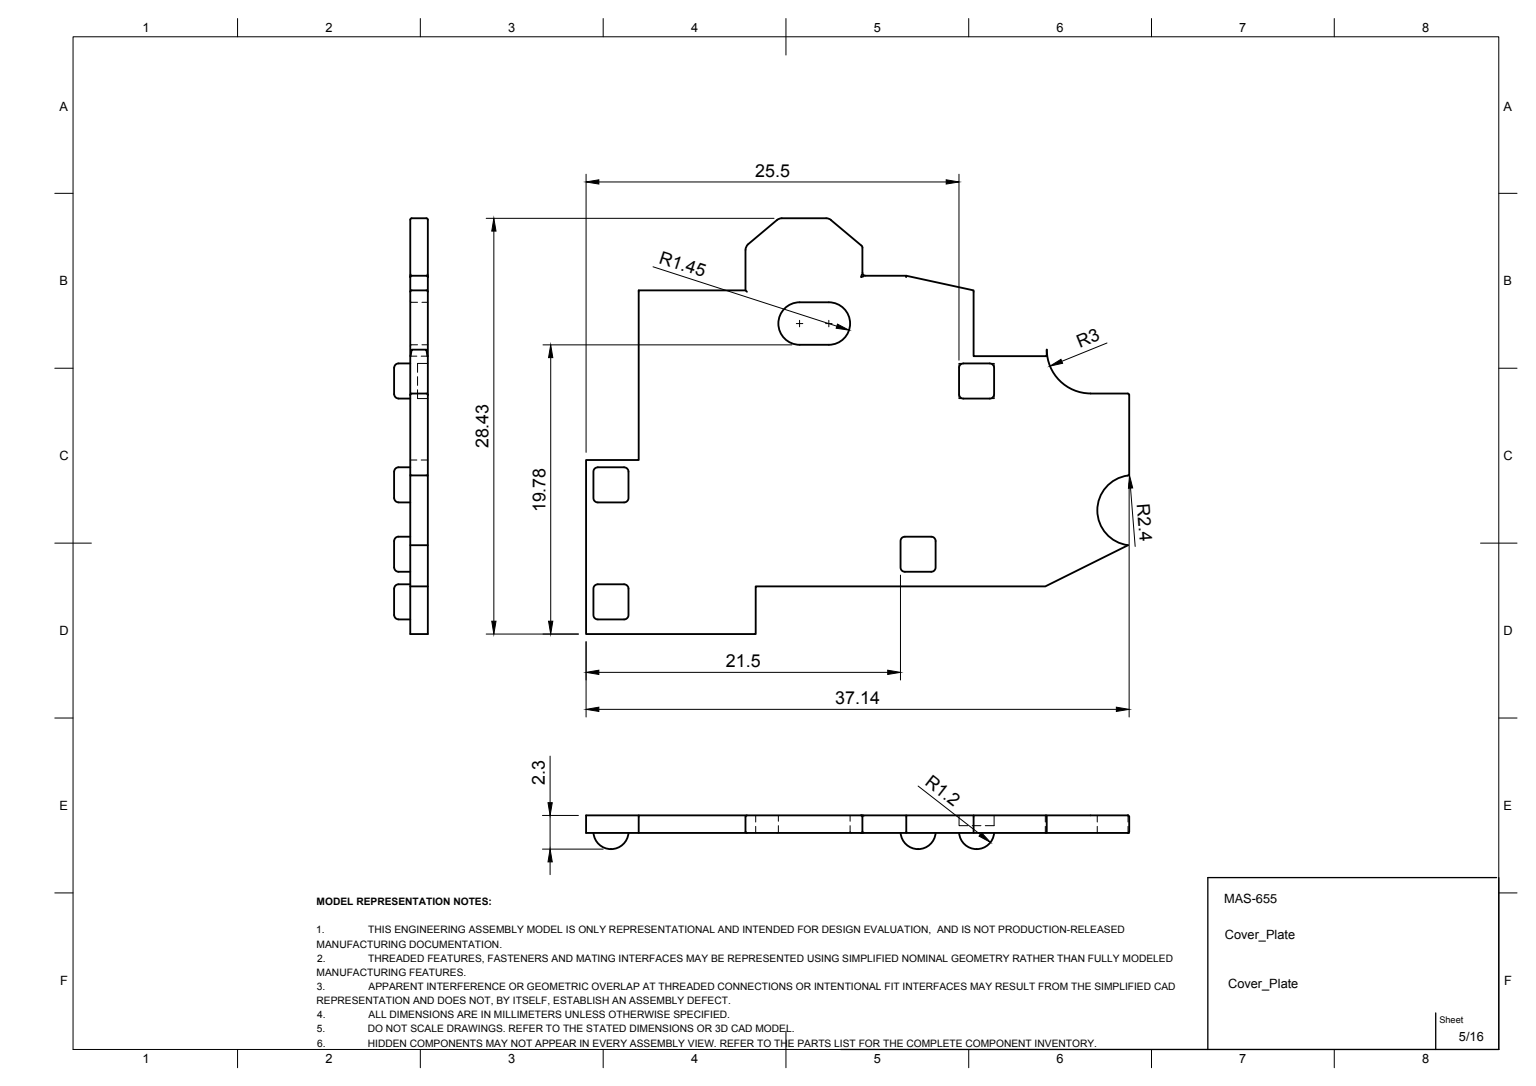
ISO-10303-21;
HEADER;
FILE_DESCRIPTION((''),'2;1');
FILE_NAME('Cover_Plate.step','2026-10-09T11:34:15-07:00',(''),(''),'','','');
FILE_SCHEMA (('AUTOMOTIVE_DESIGN { 1 0 10303 214 3 1 1 }'));
ENDSEC;
DATA;
#10=MECHANICAL_DESIGN_GEOMETRIC_PRESENTATION_REPRESENTATION('',(#632),#117170);
#95=(
BOUNDED_SURFACE()
B_SPLINE_SURFACE(2,2,((#87159,#87160,#87161),(#87162,#87163,#87164),(#87165,
#87166,#87167)),.UNSPECIFIED.,.F.,.F.,.F.)
B_SPLINE_SURFACE_WITH_KNOTS((3,3),(3,3),(2.9656421913598E-12,1.57079632680175),
(-2.44346095279454,-1.57079632680019),.UNSPECIFIED.)
GEOMETRIC_REPRESENTATION_ITEM()
RATIONAL_B_SPLINE_SURFACE(((1.,0.906307787037244,1.),(0.707106781185325,
0.640856382055101,0.707106781185325),(1.,0.906307787037244,1.)))
REPRESENTATION_ITEM('')
SURFACE()
) ;
#96=(
BOUNDED_SURFACE()
B_SPLINE_SURFACE(2,2,((#87171,#87172,#87173),(#87174,#87175,#87176),(#87177,
#87178,#87179)),.UNSPECIFIED.,.F.,.F.,.F.)
B_SPLINE_SURFACE_WITH_KNOTS((3,3),(3,3),(-1.5707963267996,-4.58626074717158E-12),
(-2.44346095281538,-1.57079632678052),.UNSPECIFIED.)
GEOMETRIC_REPRESENTATION_ITEM()
RATIONAL_B_SPLINE_SURFACE(((1.,0.906307787028686,1.),(0.707106781186676,
0.640856382050274,0.707106781186676),(1.,0.906307787028686,1.)))
REPRESENTATION_ITEM('')
SURFACE()
) ;
#269=ELLIPSE('',#51771,0.141421356237322,0.1) ;
#270=ELLIPSE('',#51774,0.141421356237322,0.1) ;
#271=ELLIPSE('',#51814,0.31622776601682,0.0999999999999979) ;
#272=ELLIPSE('',#51815,0.31622776601682,0.0999999999999979) ;
#273=ELLIPSE('',#51816,0.316227766016848,0.0999999999999979) ;
#274=ELLIPSE('',#51817,0.316227766016848,0.0999999999999979) ;
#275=ELLIPSE('',#51820,0.316227766016848,0.0999999999999979) ;
#276=ELLIPSE('',#51821,0.316227766016848,0.0999999999999979) ;
#277=ELLIPSE('',#51822,0.316227766016837,0.0999999999999979) ;
#278=ELLIPSE('',#51823,0.316227766016837,0.0999999999999979) ;
#279=ELLIPSE('',#51826,0.100574612243464,0.1) ;
#280=ELLIPSE('',#51856,0.102331928648948,0.1) ;
#281=ELLIPSE('',#51857,0.10057461224346,0.1) ;
#282=ELLIPSE('',#51862,0.102331928648948,0.1) ;
#590=SHAPE_REPRESENTATION_RELATIONSHIP('SRR','None',#117245,#611) ;
#611=ADVANCED_BREP_SHAPE_REPRESENTATION('',(#653),#117153) ;
#632=STYLED_ITEM('',(#117355),#653) ;
#653=MANIFOLD_SOLID_BREP('Body1',#49061) ;
#722=FACE_BOUND('',#15126,.T.) ;
#723=FACE_BOUND('',#15127,.T.) ;
#724=FACE_BOUND('',#15128,.T.) ;
#725=FACE_BOUND('',#15129,.T.) ;
#726=FACE_BOUND('',#15130,.T.) ;
#727=FACE_BOUND('',#15135,.T.) ;
#728=FACE_BOUND('',#15136,.T.) ;
#1127=B_SPLINE_CURVE_WITH_KNOTS('',3,(#86615,#86616,#86617,#86618,#86619,
#86620,#86621,#86622,#86623,#86624),.UNSPECIFIED.,.F.,.F.,(4,2,2,2,4),(-0.0453895164641597,
-0.0415954731675521,-0.0378014298709444,-0.0340366298274179,-0.0302718297838914),
 .UNSPECIFIED.) ;
#1128=B_SPLINE_CURVE_WITH_KNOTS('',3,(#86641,#86642,#86643,#86644,#86645,
#86646,#86647,#86648,#86649,#86650),.UNSPECIFIED.,.F.,.F.,(4,2,2,2,4),(-0.0302718297838915,
-0.0265011188029211,-0.0227304078219508,-0.0189422746940918,-0.0151541415662328),
 .UNSPECIFIED.) ;
#1129=B_SPLINE_CURVE_WITH_KNOTS('',3,(#86717,#86718,#86719,#86720,#86721,
#86722,#86723,#86724,#86725,#86726),.UNSPECIFIED.,.F.,.F.,(4,2,2,2,4),(0.13378524314305,
0.14497374491656,0.1561177263117,0.167229804836174,0.17832206951723),
 .UNSPECIFIED.) ;
#1130=B_SPLINE_CURVE_WITH_KNOTS('',3,(#86730,#86731,#86732,#86733,#86734,
#86735,#86736,#86737,#86738,#86739),.UNSPECIFIED.,.F.,.F.,(4,2,2,2,4),(0.,
0.0110922646810569,0.0222043432055302,0.0333483246006708,0.0445368263741803),
 .UNSPECIFIED.) ;
#1131=B_SPLINE_CURVE_WITH_KNOTS('',3,(#86743,#86744,#86745,#86746,#86747,
#86748,#86749,#86750,#86751,#86752),.UNSPECIFIED.,.F.,.F.,(4,2,2,2,4),(0.13378524314305,
0.14497374491656,0.1561177263117,0.167229804836174,0.17832206951723),
 .UNSPECIFIED.) ;
#1132=B_SPLINE_CURVE_WITH_KNOTS('',3,(#86756,#86757,#86758,#86759,#86760,
#86761,#86762,#86763,#86764,#86765),.UNSPECIFIED.,.F.,.F.,(4,2,2,2,4),(0.,
0.0110922646810569,0.0222043432055302,0.0333483246006708,0.0445368263741803),
 .UNSPECIFIED.) ;
#1133=B_SPLINE_CURVE_WITH_KNOTS('',3,(#86771,#86772,#86773,#86774,#86775,
#86776,#86777,#86778,#86779,#86780),.UNSPECIFIED.,.F.,.F.,(4,2,2,2,4),(0.,
0.0110922646810569,0.0222043432055302,0.0333483246006708,0.0445368263741803),
 .UNSPECIFIED.) ;
#1134=B_SPLINE_CURVE_WITH_KNOTS('',3,(#86784,#86785,#86786,#86787,#86788,
#86789,#86790,#86791,#86792,#86793),.UNSPECIFIED.,.F.,.F.,(4,2,2,2,4),(0.133785243143047,
0.144973744916557,0.156117726311698,0.167229804836173,0.17832206951723),
 .UNSPECIFIED.) ;
#1135=B_SPLINE_CURVE_WITH_KNOTS('',3,(#86797,#86798,#86799,#86800,#86801,
#86802,#86803,#86804,#86805,#86806),.UNSPECIFIED.,.F.,.F.,(4,2,2,2,4),(0.,
0.0110922646810577,0.022204343205532,0.0333483246006734,0.0445368263741838),
 .UNSPECIFIED.) ;
#1136=B_SPLINE_CURVE_WITH_KNOTS('',3,(#86809,#86810,#86811,#86812,#86813,
#86814,#86815,#86816,#86817,#86818),.UNSPECIFIED.,.F.,.F.,(4,2,2,2,4),(0.13378524314305,
0.14497374491656,0.1561177263117,0.167229804836174,0.17832206951723),
 .UNSPECIFIED.) ;
#1137=B_SPLINE_CURVE_WITH_KNOTS('',3,(#86823,#86824,#86825,#86826,#86827,
#86828,#86829,#86830,#86831,#86832),.UNSPECIFIED.,.F.,.F.,(4,2,2,2,4),(0.,
0.0110922646810577,0.022204343205532,0.0333483246006734,0.0445368263741838),
 .UNSPECIFIED.) ;
#1138=B_SPLINE_CURVE_WITH_KNOTS('',3,(#86836,#86837,#86838,#86839,#86840,
#86841,#86842,#86843,#86844,#86845),.UNSPECIFIED.,.F.,.F.,(4,2,2,2,4),(0.13378524314305,
0.14497374491656,0.1561177263117,0.167229804836174,0.17832206951723),
 .UNSPECIFIED.) ;
#1139=B_SPLINE_CURVE_WITH_KNOTS('',3,(#86849,#86850,#86851,#86852,#86853,
#86854,#86855,#86856,#86857,#86858),.UNSPECIFIED.,.F.,.F.,(4,2,2,2,4),(0.,
0.0110922646810569,0.0222043432055302,0.0333483246006708,0.0445368263741803),
 .UNSPECIFIED.) ;
#1140=B_SPLINE_CURVE_WITH_KNOTS('',3,(#86861,#86862,#86863,#86864,#86865,
#86866,#86867,#86868,#86869,#86870),.UNSPECIFIED.,.F.,.F.,(4,2,2,2,4),(0.133785243143047,
0.144973744916557,0.156117726311698,0.167229804836173,0.17832206951723),
 .UNSPECIFIED.) ;
#1141=B_SPLINE_CURVE_WITH_KNOTS('',3,(#86875,#86876,#86877,#86878,#86879,
#86880,#86881,#86882,#86883,#86884),.UNSPECIFIED.,.F.,.F.,(4,2,2,2,4),(0.,
0.0110922646810569,0.0222043432055302,0.0333483246006708,0.0445368263741803),
 .UNSPECIFIED.) ;
#1142=B_SPLINE_CURVE_WITH_KNOTS('',3,(#86888,#86889,#86890,#86891,#86892,
#86893,#86894,#86895,#86896,#86897),.UNSPECIFIED.,.F.,.F.,(4,2,2,2,4),(0.133785243143047,
0.144973744916557,0.156117726311698,0.167229804836173,0.17832206951723),
 .UNSPECIFIED.) ;
#1143=B_SPLINE_CURVE_WITH_KNOTS('',3,(#86901,#86902,#86903,#86904,#86905,
#86906,#86907,#86908,#86909,#86910),.UNSPECIFIED.,.F.,.F.,(4,2,2,2,4),(0.,
0.0110922646810577,0.022204343205532,0.0333483246006734,0.0445368263741838),
 .UNSPECIFIED.) ;
#1144=B_SPLINE_CURVE_WITH_KNOTS('',3,(#86913,#86914,#86915,#86916,#86917,
#86918,#86919,#86920,#86921,#86922),.UNSPECIFIED.,.F.,.F.,(4,2,2,2,4),(0.13378524314305,
0.14497374491656,0.1561177263117,0.167229804836174,0.17832206951723),
 .UNSPECIFIED.) ;
#1145=B_SPLINE_CURVE_WITH_KNOTS('',3,(#87209,#87210,#87211,#87212,#87213,
#87214),.UNSPECIFIED.,.F.,.F.,(4,2,4),(0.0376778444829456,0.0409098759506884,
0.0446641096906363),.UNSPECIFIED.) ;
#1146=B_SPLINE_CURVE_WITH_KNOTS('',3,(#87217,#87218,#87219,#87220),
 .UNSPECIFIED.,.F.,.F.,(4,4),(0.,0.0422101666362959),.UNSPECIFIED.) ;
#1147=B_SPLINE_CURVE_WITH_KNOTS('',3,(#87225,#87226,#87227,#87228),
 .UNSPECIFIED.,.F.,.F.,(4,4),(-0.0422101666362958,0.),.UNSPECIFIED.) ;
#1148=B_SPLINE_CURVE_WITH_KNOTS('',3,(#87235,#87236,#87237,#87238,#87239,
#87240),.UNSPECIFIED.,.F.,.F.,(4,2,4),(0.0148851463516941,0.0186393800916421,
0.021871411559383),.UNSPECIFIED.) ;
#1989=B_SPLINE_SURFACE_WITH_KNOTS('',3,3,((#87076,#87077,#87078,#87079,
#87080),(#87081,#87082,#87083,#87084,#87085),(#87086,#87087,#87088,#87089,
#87090),(#87091,#87092,#87093,#87094,#87095),(#87096,#87097,#87098,#87099,
#87100)),.UNSPECIFIED.,.F.,.F.,.F.,(4,1,4),(4,1,4),(-0.000337535876093274,
0.5,1.00033753587942),(-1.5707963267949,-0.897597901025655,0.000337535879419949),
 .UNSPECIFIED.) ;
#1990=B_SPLINE_SURFACE_WITH_KNOTS('',3,3,((#87116,#87117,#87118,#87119,
#87120),(#87121,#87122,#87123,#87124,#87125),(#87126,#87127,#87128,#87129,
#87130),(#87131,#87132,#87133,#87134,#87135),(#87136,#87137,#87138,#87139,
#87140)),.UNSPECIFIED.,.F.,.F.,.F.,(4,1,4),(4,1,4),(-0.000337608092631786,
0.5,1.00033760812633),(-1.5707963267949,-0.897597901025655,0.000337608126388777),
 .UNSPECIFIED.) ;
#2193=SPHERICAL_SURFACE('',#51742,0.1) ;
#2194=SPHERICAL_SURFACE('',#51744,0.1) ;
#2435=PLANE('',#51746) ;
#2436=PLANE('',#51757) ;
#2437=PLANE('',#51760) ;
#2438=PLANE('',#51775) ;
#2439=PLANE('',#51785) ;
#2440=PLANE('',#51799) ;
#2441=PLANE('',#51810) ;
#2442=PLANE('',#51824) ;
#2443=PLANE('',#51834) ;
#2444=PLANE('',#51846) ;
#2445=PLANE('',#51849) ;
#2446=PLANE('',#51852) ;
#2447=PLANE('',#51854) ;
#2448=PLANE('',#51861) ;
#2449=PLANE('',#51863) ;
#2450=PLANE('',#51864) ;
#2451=PLANE('',#51876) ;
#2452=PLANE('',#51886) ;
#2453=PLANE('',#51896) ;
#2454=PLANE('',#51906) ;
#2455=PLANE('',#51916) ;
#2456=PLANE('',#51926) ;
#2457=PLANE('',#51936) ;
#2458=PLANE('',#51946) ;
#2459=PLANE('',#51948) ;
#2460=PLANE('',#51951) ;
#2461=PLANE('',#51954) ;
#2462=PLANE('',#51957) ;
#2463=PLANE('',#51959) ;
#2464=PLANE('',#51960) ;
#2465=PLANE('',#51961) ;
#2466=PLANE('',#51963) ;
#2467=PLANE('',#51964) ;
#2468=PLANE('',#51966) ;
#2469=PLANE('',#51967) ;
#2470=PLANE('',#51968) ;
#2471=PLANE('',#51969) ;
#2472=PLANE('',#51970) ;
#2473=PLANE('',#51971) ;
#2474=PLANE('',#51972) ;
#2475=PLANE('',#51973) ;
#4105=LINE('',#86626,#7319) ;
#4106=LINE('',#86629,#7320) ;
#4107=LINE('',#86634,#7321) ;
#4108=LINE('',#86637,#7322) ;
#4109=LINE('',#86652,#7323) ;
#4110=LINE('',#86654,#7324) ;
#4111=LINE('',#86661,#7325) ;
#4112=LINE('',#86665,#7326) ;
#4113=LINE('',#86667,#7327) ;
#4114=LINE('',#86669,#7328) ;
#4115=LINE('',#86671,#7329) ;
#4116=LINE('',#86673,#7330) ;
#4117=LINE('',#86677,#7331) ;
#4118=LINE('',#86681,#7332) ;
#4119=LINE('',#86685,#7333) ;
#4120=LINE('',#86689,#7334) ;
#4121=LINE('',#86691,#7335) ;
#4122=LINE('',#86693,#7336) ;
#4123=LINE('',#86695,#7337) ;
#4124=LINE('',#86697,#7338) ;
#4125=LINE('',#86699,#7339) ;
#4126=LINE('',#86701,#7340) ;
#4127=LINE('',#86703,#7341) ;
#4128=LINE('',#86705,#7342) ;
#4129=LINE('',#86709,#7343) ;
#4130=LINE('',#86713,#7344) ;
#4131=LINE('',#86728,#7345) ;
#4132=LINE('',#86741,#7346) ;
#4133=LINE('',#86754,#7347) ;
#4134=LINE('',#86766,#7348) ;
#4135=LINE('',#86769,#7349) ;
#4136=LINE('',#86782,#7350) ;
#4137=LINE('',#86795,#7351) ;
#4138=LINE('',#86808,#7352) ;
#4139=LINE('',#86821,#7353) ;
#4140=LINE('',#86834,#7354) ;
#4141=LINE('',#86847,#7355) ;
#4142=LINE('',#86860,#7356) ;
#4143=LINE('',#86873,#7357) ;
#4144=LINE('',#86886,#7358) ;
#4145=LINE('',#86899,#7359) ;
#4146=LINE('',#86912,#7360) ;
#4147=LINE('',#86925,#7361) ;
#4148=LINE('',#86929,#7362) ;
#4149=LINE('',#86930,#7363) ;
#4150=LINE('',#86933,#7364) ;
#4151=LINE('',#86939,#7365) ;
#4152=LINE('',#86941,#7366) ;
#4153=LINE('',#86943,#7367) ;
#4154=LINE('',#86945,#7368) ;
#4155=LINE('',#86947,#7369) ;
#4156=LINE('',#86949,#7370) ;
#4157=LINE('',#86951,#7371) ;
#4158=LINE('',#86953,#7372) ;
#4159=LINE('',#86955,#7373) ;
#4160=LINE('',#86959,#7374) ;
#4161=LINE('',#86963,#7375) ;
#4162=LINE('',#86967,#7376) ;
#4163=LINE('',#86971,#7377) ;
#4164=LINE('',#86973,#7378) ;
#4165=LINE('',#86975,#7379) ;
#4166=LINE('',#86977,#7380) ;
#4167=LINE('',#86979,#7381) ;
#4168=LINE('',#86985,#7382) ;
#4169=LINE('',#86988,#7383) ;
#4170=LINE('',#86991,#7384) ;
#4171=LINE('',#86993,#7385) ;
#4172=LINE('',#86995,#7386) ;
#4173=LINE('',#86996,#7387) ;
#4174=LINE('',#87001,#7388) ;
#4175=LINE('',#87008,#7389) ;
#4176=LINE('',#87010,#7390) ;
#4177=LINE('',#87011,#7391) ;
#4178=LINE('',#87025,#7392) ;
#4179=LINE('',#87026,#7393) ;
#4180=LINE('',#87029,#7394) ;
#4181=LINE('',#87031,#7395) ;
#4182=LINE('',#87032,#7396) ;
#4183=LINE('',#87037,#7397) ;
#4184=LINE('',#87050,#7398) ;
#4185=LINE('',#87051,#7399) ;
#4186=LINE('',#87053,#7400) ;
#4187=LINE('',#87065,#7401) ;
#4188=LINE('',#87068,#7402) ;
#4189=LINE('',#87072,#7403) ;
#4190=LINE('',#87073,#7404) ;
#4191=LINE('',#87112,#7405) ;
#4192=LINE('',#87115,#7406) ;
#4193=LINE('',#87149,#7407) ;
#4194=LINE('',#87151,#7408) ;
#4195=LINE('',#87152,#7409) ;
#4196=LINE('',#87157,#7410) ;
#4197=LINE('',#87182,#7411) ;
#4198=LINE('',#87184,#7412) ;
#4199=LINE('',#87191,#7413) ;
#4200=LINE('',#87199,#7414) ;
#4201=LINE('',#87203,#7415) ;
#4202=LINE('',#87204,#7416) ;
#4203=LINE('',#87206,#7417) ;
#4204=LINE('',#87223,#7418) ;
#4205=LINE('',#87229,#7419) ;
#4206=LINE('',#87233,#7420) ;
#4207=LINE('',#87242,#7421) ;
#4208=LINE('',#87245,#7422) ;
#4209=LINE('',#87251,#7423) ;
#4210=LINE('',#87254,#7424) ;
#4211=LINE('',#87257,#7425) ;
#4212=LINE('',#87259,#7426) ;
#4213=LINE('',#87272,#7427) ;
#4214=LINE('',#87273,#7428) ;
#4215=LINE('',#87288,#7429) ;
#4216=LINE('',#87289,#7430) ;
#4217=LINE('',#87304,#7431) ;
#4218=LINE('',#87305,#7432) ;
#4219=LINE('',#87320,#7433) ;
#4220=LINE('',#87321,#7434) ;
#4221=LINE('',#87336,#7435) ;
#4222=LINE('',#87337,#7436) ;
#4223=LINE('',#87352,#7437) ;
#4224=LINE('',#87353,#7438) ;
#4225=LINE('',#87368,#7439) ;
#4226=LINE('',#87369,#7440) ;
#4227=LINE('',#87384,#7441) ;
#4228=LINE('',#87385,#7442) ;
#4229=LINE('',#87391,#7443) ;
#4230=LINE('',#87393,#7444) ;
#4231=LINE('',#87396,#7445) ;
#4232=LINE('',#87398,#7446) ;
#4233=LINE('',#87401,#7447) ;
#4234=LINE('',#87403,#7448) ;
#4235=LINE('',#87406,#7449) ;
#4236=LINE('',#87408,#7450) ;
#4237=LINE('',#87413,#7451) ;
#4238=LINE('',#87415,#7452) ;
#4239=LINE('',#87417,#7453) ;
#4240=LINE('',#87418,#7454) ;
#4241=LINE('',#87420,#7455) ;
#4242=LINE('',#87421,#7456) ;
#4243=LINE('',#87423,#7457) ;
#4244=LINE('',#87425,#7458) ;
#4245=LINE('',#87427,#7459) ;
#4246=LINE('',#87429,#7460) ;
#4247=LINE('',#87432,#7461) ;
#4248=LINE('',#87435,#7462) ;
#4249=LINE('',#87437,#7463) ;
#4250=LINE('',#87439,#7464) ;
#4251=LINE('',#87441,#7465) ;
#4252=LINE('',#87443,#7466) ;
#7319=VECTOR('',#61022,10.) ;
#7320=VECTOR('',#61025,10.) ;
#7321=VECTOR('',#61030,10.) ;
#7322=VECTOR('',#61033,10.) ;
#7323=VECTOR('',#61036,10.) ;
#7324=VECTOR('',#61039,10.) ;
#7325=VECTOR('',#61050,10.) ;
#7326=VECTOR('',#61053,10.) ;
#7327=VECTOR('',#61054,10.) ;
#7328=VECTOR('',#61055,10.) ;
#7329=VECTOR('',#61056,10.) ;
#7330=VECTOR('',#61057,10.) ;
#7331=VECTOR('',#61060,10.) ;
#7332=VECTOR('',#61063,10.) ;
#7333=VECTOR('',#61066,10.) ;
#7334=VECTOR('',#61069,10.) ;
#7335=VECTOR('',#61070,10.) ;
#7336=VECTOR('',#61071,10.) ;
#7337=VECTOR('',#61072,10.) ;
#7338=VECTOR('',#61073,10.) ;
#7339=VECTOR('',#61074,10.) ;
#7340=VECTOR('',#61075,10.) ;
#7341=VECTOR('',#61076,10.) ;
#7342=VECTOR('',#61077,10.) ;
#7343=VECTOR('',#61080,10.) ;
#7344=VECTOR('',#61083,10.) ;
#7345=VECTOR('',#61086,10.) ;
#7346=VECTOR('',#61087,10.) ;
#7347=VECTOR('',#61088,10.) ;
#7348=VECTOR('',#61089,10.) ;
#7349=VECTOR('',#61090,10.) ;
#7350=VECTOR('',#61091,10.) ;
#7351=VECTOR('',#61092,10.) ;
#7352=VECTOR('',#61093,10.) ;
#7353=VECTOR('',#61094,10.) ;
#7354=VECTOR('',#61095,10.) ;
#7355=VECTOR('',#61096,10.) ;
#7356=VECTOR('',#61097,10.) ;
#7357=VECTOR('',#61098,10.) ;
#7358=VECTOR('',#61099,10.) ;
#7359=VECTOR('',#61100,10.) ;
#7360=VECTOR('',#61101,10.) ;
#7361=VECTOR('',#61104,10.) ;
#7362=VECTOR('',#61109,10.) ;
#7363=VECTOR('',#61110,10.) ;
#7364=VECTOR('',#61113,10.) ;
#7365=VECTOR('',#61120,10.) ;
#7366=VECTOR('',#61121,10.) ;
#7367=VECTOR('',#61122,10.) ;
#7368=VECTOR('',#61123,10.) ;
#7369=VECTOR('',#61124,10.) ;
#7370=VECTOR('',#61125,10.) ;
#7371=VECTOR('',#61126,10.) ;
#7372=VECTOR('',#61127,10.) ;
#7373=VECTOR('',#61128,10.) ;
#7374=VECTOR('',#61131,10.) ;
#7375=VECTOR('',#61134,10.) ;
#7376=VECTOR('',#61137,10.) ;
#7377=VECTOR('',#61140,10.) ;
#7378=VECTOR('',#61141,10.) ;
#7379=VECTOR('',#61142,10.) ;
#7380=VECTOR('',#61143,10.) ;
#7381=VECTOR('',#61144,10.) ;
#7382=VECTOR('',#61149,10.) ;
#7383=VECTOR('',#61152,10.) ;
#7384=VECTOR('',#61153,10.) ;
#7385=VECTOR('',#61154,10.) ;
#7386=VECTOR('',#61155,10.) ;
#7387=VECTOR('',#61156,10.) ;
#7388=VECTOR('',#61161,10.) ;
#7389=VECTOR('',#61170,10.) ;
#7390=VECTOR('',#61173,10.) ;
#7391=VECTOR('',#61174,10.) ;
#7392=VECTOR('',#61193,10.) ;
#7393=VECTOR('',#61194,10.) ;
#7394=VECTOR('',#61197,10.) ;
#7395=VECTOR('',#61198,10.) ;
#7396=VECTOR('',#61199,10.) ;
#7397=VECTOR('',#61206,10.) ;
#7398=VECTOR('',#61225,10.) ;
#7399=VECTOR('',#61226,10.) ;
#7400=VECTOR('',#61229,10.) ;
#7401=VECTOR('',#61248,10.) ;
#7402=VECTOR('',#61251,10.) ;
#7403=VECTOR('',#61256,10.) ;
#7404=VECTOR('',#61257,10.) ;
#7405=VECTOR('',#61274,10.) ;
#7406=VECTOR('',#61277,10.) ;
#7407=VECTOR('',#61288,10.) ;
#7408=VECTOR('',#61289,10.) ;
#7409=VECTOR('',#61290,10.) ;
#7410=VECTOR('',#61297,10.) ;
#7411=VECTOR('',#61308,10.) ;
#7412=VECTOR('',#61311,10.) ;
#7413=VECTOR('',#61320,10.) ;
#7414=VECTOR('',#61331,10.) ;
#7415=VECTOR('',#61338,10.) ;
#7416=VECTOR('',#61339,10.) ;
#7417=VECTOR('',#61342,10.) ;
#7418=VECTOR('',#61349,10.) ;
#7419=VECTOR('',#61350,10.) ;
#7420=VECTOR('',#61357,10.) ;
#7421=VECTOR('',#61362,10.) ;
#7422=VECTOR('',#61365,10.) ;
#7423=VECTOR('',#61376,10.) ;
#7424=VECTOR('',#61379,10.) ;
#7425=VECTOR('',#61384,10.) ;
#7426=VECTOR('',#61387,10.) ;
#7427=VECTOR('',#61404,10.) ;
#7428=VECTOR('',#61405,10.) ;
#7429=VECTOR('',#61426,10.) ;
#7430=VECTOR('',#61427,10.) ;
#7431=VECTOR('',#61448,10.) ;
#7432=VECTOR('',#61449,10.) ;
#7433=VECTOR('',#61470,10.) ;
#7434=VECTOR('',#61471,10.) ;
#7435=VECTOR('',#61492,10.) ;
#7436=VECTOR('',#61493,10.) ;
#7437=VECTOR('',#61514,10.) ;
#7438=VECTOR('',#61515,10.) ;
#7439=VECTOR('',#61536,10.) ;
#7440=VECTOR('',#61537,10.) ;
#7441=VECTOR('',#61558,10.) ;
#7442=VECTOR('',#61559,10.) ;
#7443=VECTOR('',#61570,1.2) ;
#7444=VECTOR('',#61573,1.2) ;
#7445=VECTOR('',#61578,1.2) ;
#7446=VECTOR('',#61581,1.2) ;
#7447=VECTOR('',#61586,1.2) ;
#7448=VECTOR('',#61589,1.2) ;
#7449=VECTOR('',#61594,1.2) ;
#7450=VECTOR('',#61597,1.2) ;
#7451=VECTOR('',#61602,10.) ;
#7452=VECTOR('',#61603,10.) ;
#7453=VECTOR('',#61604,10.) ;
#7454=VECTOR('',#61605,10.) ;
#7455=VECTOR('',#61608,10.) ;
#7456=VECTOR('',#61609,10.) ;
#7457=VECTOR('',#61612,10.) ;
#7458=VECTOR('',#61615,10.) ;
#7459=VECTOR('',#61618,10.) ;
#7460=VECTOR('',#61621,10.) ;
#7461=VECTOR('',#61626,10.) ;
#7462=VECTOR('',#61631,10.) ;
#7463=VECTOR('',#61634,10.) ;
#7464=VECTOR('',#61637,10.) ;
#7465=VECTOR('',#61640,10.) ;
#7466=VECTOR('',#61643,10.) ;
#9939=CYLINDRICAL_SURFACE('',#51735,0.1) ;
#9940=CYLINDRICAL_SURFACE('',#51737,0.1) ;
#9941=CYLINDRICAL_SURFACE('',#51740,0.1) ;
#9942=CYLINDRICAL_SURFACE('',#51755,0.1) ;
#9943=CYLINDRICAL_SURFACE('',#51758,0.1) ;
#9944=CYLINDRICAL_SURFACE('',#51769,0.1) ;
#9945=CYLINDRICAL_SURFACE('',#51772,0.1) ;
#9946=CYLINDRICAL_SURFACE('',#51784,0.5) ;
#9947=CYLINDRICAL_SURFACE('',#51786,0.1) ;
#9948=CYLINDRICAL_SURFACE('',#51788,0.1) ;
#9949=CYLINDRICAL_SURFACE('',#51797,0.5) ;
#9950=CYLINDRICAL_SURFACE('',#51798,0.1) ;
#9951=CYLINDRICAL_SURFACE('',#51807,0.5) ;
#9952=CYLINDRICAL_SURFACE('',#51808,0.1) ;
#9953=CYLINDRICAL_SURFACE('',#51811,0.1) ;
#9954=CYLINDRICAL_SURFACE('',#51818,0.2) ;
#9955=CYLINDRICAL_SURFACE('',#51825,0.1) ;
#9956=CYLINDRICAL_SURFACE('',#51827,0.1) ;
#9957=CYLINDRICAL_SURFACE('',#51832,0.2) ;
#9958=CYLINDRICAL_SURFACE('',#51833,0.1) ;
#9959=CYLINDRICAL_SURFACE('',#51835,0.1) ;
#9960=CYLINDRICAL_SURFACE('',#51841,0.1) ;
#9961=CYLINDRICAL_SURFACE('',#51845,1.45266329058736) ;
#9962=CYLINDRICAL_SURFACE('',#51850,3.) ;
#9963=CYLINDRICAL_SURFACE('',#51855,0.1) ;
#9964=CYLINDRICAL_SURFACE('',#51858,0.1) ;
#9965=CYLINDRICAL_SURFACE('',#51859,0.1) ;
#9966=CYLINDRICAL_SURFACE('',#51860,0.1) ;
#9967=CYLINDRICAL_SURFACE('',#51865,0.1) ;
#9968=CYLINDRICAL_SURFACE('',#51866,0.1) ;
#9969=CYLINDRICAL_SURFACE('',#51871,0.3) ;
#9970=CYLINDRICAL_SURFACE('',#51881,0.3) ;
#9971=CYLINDRICAL_SURFACE('',#51891,0.3) ;
#9972=CYLINDRICAL_SURFACE('',#51901,0.3) ;
#9973=CYLINDRICAL_SURFACE('',#51911,0.3) ;
#9974=CYLINDRICAL_SURFACE('',#51921,0.3) ;
#9975=CYLINDRICAL_SURFACE('',#51931,0.3) ;
#9976=CYLINDRICAL_SURFACE('',#51941,0.3) ;
#9977=CYLINDRICAL_SURFACE('',#51947,1.19999999999999) ;
#9978=CYLINDRICAL_SURFACE('',#51949,1.19999999999999) ;
#9979=CYLINDRICAL_SURFACE('',#51950,1.19999999999999) ;
#9980=CYLINDRICAL_SURFACE('',#51952,1.19999999999999) ;
#9981=CYLINDRICAL_SURFACE('',#51953,1.19999999999999) ;
#9982=CYLINDRICAL_SURFACE('',#51955,1.19999999999999) ;
#9983=CYLINDRICAL_SURFACE('',#51956,1.19999999999999) ;
#9984=CYLINDRICAL_SURFACE('',#51958,1.19999999999999) ;
#9985=CYLINDRICAL_SURFACE('',#51962,2.4) ;
#9986=CYLINDRICAL_SURFACE('',#51965,1.45266329058736) ;
#11976=FACE_OUTER_BOUND('',#15120,.T.) ;
#11977=FACE_OUTER_BOUND('',#15121,.T.) ;
#11978=FACE_OUTER_BOUND('',#15122,.T.) ;
#11979=FACE_OUTER_BOUND('',#15123,.T.) ;
#11980=FACE_OUTER_BOUND('',#15124,.T.) ;
#11981=FACE_OUTER_BOUND('',#15125,.T.) ;
#11982=FACE_OUTER_BOUND('',#15131,.T.) ;
#11983=FACE_OUTER_BOUND('',#15132,.T.) ;
#11984=FACE_OUTER_BOUND('',#15133,.T.) ;
#11985=FACE_OUTER_BOUND('',#15134,.T.) ;
#11986=FACE_OUTER_BOUND('',#15137,.T.) ;
#11987=FACE_OUTER_BOUND('',#15138,.T.) ;
#11988=FACE_OUTER_BOUND('',#15139,.T.) ;
#11989=FACE_OUTER_BOUND('',#15140,.T.) ;
#11990=FACE_OUTER_BOUND('',#15141,.T.) ;
#11991=FACE_OUTER_BOUND('',#15142,.T.) ;
#11992=FACE_OUTER_BOUND('',#15143,.T.) ;
#11993=FACE_OUTER_BOUND('',#15144,.T.) ;
#11994=FACE_OUTER_BOUND('',#15145,.T.) ;
#11995=FACE_OUTER_BOUND('',#15146,.T.) ;
#11996=FACE_OUTER_BOUND('',#15147,.T.) ;
#11997=FACE_OUTER_BOUND('',#15148,.T.) ;
#11998=FACE_OUTER_BOUND('',#15149,.T.) ;
#11999=FACE_OUTER_BOUND('',#15150,.T.) ;
#12000=FACE_OUTER_BOUND('',#15151,.T.) ;
#12001=FACE_OUTER_BOUND('',#15152,.T.) ;
#12002=FACE_OUTER_BOUND('',#15153,.T.) ;
#12003=FACE_OUTER_BOUND('',#15154,.T.) ;
#12004=FACE_OUTER_BOUND('',#15155,.T.) ;
#12005=FACE_OUTER_BOUND('',#15156,.T.) ;
#12006=FACE_OUTER_BOUND('',#15157,.T.) ;
#12007=FACE_OUTER_BOUND('',#15158,.T.) ;
#12008=FACE_OUTER_BOUND('',#15159,.T.) ;
#12009=FACE_OUTER_BOUND('',#15160,.T.) ;
#12010=FACE_OUTER_BOUND('',#15161,.T.) ;
#12011=FACE_OUTER_BOUND('',#15162,.T.) ;
#12012=FACE_OUTER_BOUND('',#15163,.T.) ;
#12013=FACE_OUTER_BOUND('',#15164,.T.) ;
#12014=FACE_OUTER_BOUND('',#15165,.T.) ;
#12015=FACE_OUTER_BOUND('',#15166,.T.) ;
#12016=FACE_OUTER_BOUND('',#15167,.T.) ;
#12017=FACE_OUTER_BOUND('',#15168,.T.) ;
#12018=FACE_OUTER_BOUND('',#15169,.T.) ;
#12019=FACE_OUTER_BOUND('',#15170,.T.) ;
#12020=FACE_OUTER_BOUND('',#15171,.T.) ;
#12021=FACE_OUTER_BOUND('',#15172,.T.) ;
#12022=FACE_OUTER_BOUND('',#15173,.T.) ;
#12023=FACE_OUTER_BOUND('',#15174,.T.) ;
#12024=FACE_OUTER_BOUND('',#15175,.T.) ;
#12025=FACE_OUTER_BOUND('',#15176,.T.) ;
#12026=FACE_OUTER_BOUND('',#15177,.T.) ;
#12027=FACE_OUTER_BOUND('',#15178,.T.) ;
#12028=FACE_OUTER_BOUND('',#15179,.T.) ;
#12029=FACE_OUTER_BOUND('',#15180,.T.) ;
#12030=FACE_OUTER_BOUND('',#15181,.T.) ;
#12031=FACE_OUTER_BOUND('',#15182,.T.) ;
#12032=FACE_OUTER_BOUND('',#15183,.T.) ;
#12033=FACE_OUTER_BOUND('',#15184,.T.) ;
#12034=FACE_OUTER_BOUND('',#15185,.T.) ;
#12035=FACE_OUTER_BOUND('',#15186,.T.) ;
#12036=FACE_OUTER_BOUND('',#15187,.T.) ;
#12037=FACE_OUTER_BOUND('',#15188,.T.) ;
#12038=FACE_OUTER_BOUND('',#15189,.T.) ;
#12039=FACE_OUTER_BOUND('',#15190,.T.) ;
#12040=FACE_OUTER_BOUND('',#15191,.T.) ;
#12041=FACE_OUTER_BOUND('',#15192,.T.) ;
#12042=FACE_OUTER_BOUND('',#15193,.T.) ;
#12043=FACE_OUTER_BOUND('',#15194,.T.) ;
#12044=FACE_OUTER_BOUND('',#15195,.T.) ;
#12045=FACE_OUTER_BOUND('',#15196,.T.) ;
#12046=FACE_OUTER_BOUND('',#15197,.T.) ;
#12047=FACE_OUTER_BOUND('',#15198,.T.) ;
#12048=FACE_OUTER_BOUND('',#15199,.T.) ;
#12049=FACE_OUTER_BOUND('',#15200,.T.) ;
#12050=FACE_OUTER_BOUND('',#15201,.T.) ;
#12051=FACE_OUTER_BOUND('',#15202,.T.) ;
#12052=FACE_OUTER_BOUND('',#15203,.T.) ;
#12053=FACE_OUTER_BOUND('',#15204,.T.) ;
#12054=FACE_OUTER_BOUND('',#15205,.T.) ;
#12055=FACE_OUTER_BOUND('',#15206,.T.) ;
#12056=FACE_OUTER_BOUND('',#15207,.T.) ;
#12057=FACE_OUTER_BOUND('',#15208,.T.) ;
#12058=FACE_OUTER_BOUND('',#15209,.T.) ;
#12059=FACE_OUTER_BOUND('',#15210,.T.) ;
#12060=FACE_OUTER_BOUND('',#15211,.T.) ;
#12061=FACE_OUTER_BOUND('',#15212,.T.) ;
#12062=FACE_OUTER_BOUND('',#15213,.T.) ;
#12063=FACE_OUTER_BOUND('',#15214,.T.) ;
#12064=FACE_OUTER_BOUND('',#15215,.T.) ;
#12065=FACE_OUTER_BOUND('',#15216,.T.) ;
#12066=FACE_OUTER_BOUND('',#15217,.T.) ;
#12067=FACE_OUTER_BOUND('',#15218,.T.) ;
#12068=FACE_OUTER_BOUND('',#15219,.T.) ;
#12069=FACE_OUTER_BOUND('',#15220,.T.) ;
#12070=FACE_OUTER_BOUND('',#15221,.T.) ;
#12071=FACE_OUTER_BOUND('',#15222,.T.) ;
#12072=FACE_OUTER_BOUND('',#15223,.T.) ;
#12073=FACE_OUTER_BOUND('',#15224,.T.) ;
#12074=FACE_OUTER_BOUND('',#15225,.T.) ;
#12075=FACE_OUTER_BOUND('',#15226,.T.) ;
#12076=FACE_OUTER_BOUND('',#15227,.T.) ;
#12077=FACE_OUTER_BOUND('',#15228,.T.) ;
#12078=FACE_OUTER_BOUND('',#15229,.T.) ;
#12079=FACE_OUTER_BOUND('',#15230,.T.) ;
#12080=FACE_OUTER_BOUND('',#15231,.T.) ;
#12081=FACE_OUTER_BOUND('',#15232,.T.) ;
#12082=FACE_OUTER_BOUND('',#15233,.T.) ;
#12083=FACE_OUTER_BOUND('',#15234,.T.) ;
#12084=FACE_OUTER_BOUND('',#15235,.T.) ;
#12085=FACE_OUTER_BOUND('',#15236,.T.) ;
#12086=FACE_OUTER_BOUND('',#15237,.T.) ;
#12087=FACE_OUTER_BOUND('',#15238,.T.) ;
#12088=FACE_OUTER_BOUND('',#15239,.T.) ;
#12089=FACE_OUTER_BOUND('',#15240,.T.) ;
#12090=FACE_OUTER_BOUND('',#15241,.T.) ;
#12091=FACE_OUTER_BOUND('',#15242,.T.) ;
#12092=FACE_OUTER_BOUND('',#15243,.T.) ;
#12093=FACE_OUTER_BOUND('',#15244,.T.) ;
#12094=FACE_OUTER_BOUND('',#15245,.T.) ;
#12095=FACE_OUTER_BOUND('',#15246,.T.) ;
#12096=FACE_OUTER_BOUND('',#15247,.T.) ;
#15120=EDGE_LOOP('',(#36666,#36667,#36668,#36669)) ;
#15121=EDGE_LOOP('',(#36670,#36671,#36672,#36673)) ;
#15122=EDGE_LOOP('',(#36674,#36675,#36676,#36677)) ;
#15123=EDGE_LOOP('',(#36678,#36679,#36680)) ;
#15124=EDGE_LOOP('',(#36681,#36682,#36683)) ;
#15125=EDGE_LOOP('',(#36684,#36685,#36686,#36687,#36688,#36689,#36690,#36691,
#36692,#36693,#36694,#36695,#36696,#36697,#36698,#36699,#36700,#36701,#36702,
#36703,#36704,#36705,#36706,#36707,#36708)) ;
#15126=EDGE_LOOP('',(#36709,#36710,#36711,#36712)) ;
#15127=EDGE_LOOP('',(#36713,#36714,#36715,#36716,#36717,#36718,#36719,#36720)) ;
#15128=EDGE_LOOP('',(#36721,#36722,#36723,#36724,#36725,#36726,#36727,#36728)) ;
#15129=EDGE_LOOP('',(#36729,#36730,#36731,#36732,#36733,#36734,#36735,#36736)) ;
#15130=EDGE_LOOP('',(#36737,#36738,#36739,#36740,#36741,#36742,#36743,#36744)) ;
#15131=EDGE_LOOP('',(#36745,#36746,#36747,#36748)) ;
#15132=EDGE_LOOP('',(#36749,#36750,#36751,#36752)) ;
#15133=EDGE_LOOP('',(#36753,#36754,#36755,#36756)) ;
#15134=EDGE_LOOP('',(#36757,#36758,#36759,#36760,#36761,#36762,#36763,#36764,
#36765,#36766,#36767,#36768,#36769,#36770,#36771,#36772,#36773,#36774,#36775,
#36776,#36777,#36778,#36779,#36780,#36781)) ;
#15135=EDGE_LOOP('',(#36782,#36783,#36784,#36785)) ;
#15136=EDGE_LOOP('',(#36786,#36787,#36788,#36789)) ;
#15137=EDGE_LOOP('',(#36790,#36791,#36792,#36793)) ;
#15138=EDGE_LOOP('',(#36794,#36795,#36796,#36797)) ;
#15139=EDGE_LOOP('',(#36798,#36799,#36800,#36801)) ;
#15140=EDGE_LOOP('',(#36802,#36803,#36804,#36805)) ;
#15141=EDGE_LOOP('',(#36806,#36807,#36808,#36809)) ;
#15142=EDGE_LOOP('',(#36810,#36811,#36812,#36813)) ;
#15143=EDGE_LOOP('',(#36814,#36815,#36816,#36817)) ;
#15144=EDGE_LOOP('',(#36818,#36819,#36820,#36821)) ;
#15145=EDGE_LOOP('',(#36822,#36823,#36824,#36825)) ;
#15146=EDGE_LOOP('',(#36826,#36827,#36828,#36829)) ;
#15147=EDGE_LOOP('',(#36830,#36831,#36832,#36833)) ;
#15148=EDGE_LOOP('',(#36834,#36835,#36836,#36837)) ;
#15149=EDGE_LOOP('',(#36838,#36839,#36840,#36841)) ;
#15150=EDGE_LOOP('',(#36842,#36843,#36844,#36845)) ;
#15151=EDGE_LOOP('',(#36846,#36847,#36848,#36849)) ;
#15152=EDGE_LOOP('',(#36850,#36851,#36852,#36853)) ;
#15153=EDGE_LOOP('',(#36854,#36855,#36856,#36857)) ;
#15154=EDGE_LOOP('',(#36858,#36859,#36860,#36861)) ;
#15155=EDGE_LOOP('',(#36862,#36863,#36864,#36865)) ;
#15156=EDGE_LOOP('',(#36866,#36867,#36868,#36869)) ;
#15157=EDGE_LOOP('',(#36870,#36871,#36872,#36873,#36874)) ;
#15158=EDGE_LOOP('',(#36875,#36876,#36877,#36878)) ;
#15159=EDGE_LOOP('',(#36879,#36880,#36881,#36882,#36883)) ;
#15160=EDGE_LOOP('',(#36884,#36885,#36886,#36887)) ;
#15161=EDGE_LOOP('',(#36888,#36889,#36890,#36891,#36892)) ;
#15162=EDGE_LOOP('',(#36893,#36894,#36895,#36896,#36897)) ;
#15163=EDGE_LOOP('',(#36898,#36899,#36900,#36901)) ;
#15164=EDGE_LOOP('',(#36902,#36903,#36904,#36905)) ;
#15165=EDGE_LOOP('',(#36906,#36907,#36908,#36909)) ;
#15166=EDGE_LOOP('',(#36910,#36911,#36912,#36913,#36914)) ;
#15167=EDGE_LOOP('',(#36915,#36916,#36917,#36918)) ;
#15168=EDGE_LOOP('',(#36919,#36920,#36921,#36922)) ;
#15169=EDGE_LOOP('',(#36923,#36924,#36925,#36926)) ;
#15170=EDGE_LOOP('',(#36927,#36928,#36929,#36930)) ;
#15171=EDGE_LOOP('',(#36931,#36932,#36933,#36934)) ;
#15172=EDGE_LOOP('',(#36935,#36936,#36937,#36938)) ;
#15173=EDGE_LOOP('',(#36939,#36940,#36941,#36942)) ;
#15174=EDGE_LOOP('',(#36943,#36944,#36945,#36946,#36947)) ;
#15175=EDGE_LOOP('',(#36948,#36949,#36950,#36951)) ;
#15176=EDGE_LOOP('',(#36952,#36953,#36954,#36955)) ;
#15177=EDGE_LOOP('',(#36956,#36957,#36958,#36959)) ;
#15178=EDGE_LOOP('',(#36960,#36961,#36962,#36963,#36964)) ;
#15179=EDGE_LOOP('',(#36965,#36966,#36967,#36968,#36969,#36970)) ;
#15180=EDGE_LOOP('',(#36971,#36972,#36973,#36974)) ;
#15181=EDGE_LOOP('',(#36975,#36976,#36977,#36978,#36979)) ;
#15182=EDGE_LOOP('',(#36980,#36981,#36982,#36983)) ;
#15183=EDGE_LOOP('',(#36984,#36985,#36986,#36987)) ;
#15184=EDGE_LOOP('',(#36988,#36989,#36990,#36991,#36992,#36993)) ;
#15185=EDGE_LOOP('',(#36994,#36995,#36996,#36997)) ;
#15186=EDGE_LOOP('',(#36998,#36999,#37000,#37001)) ;
#15187=EDGE_LOOP('',(#37002,#37003,#37004,#37005)) ;
#15188=EDGE_LOOP('',(#37006,#37007,#37008,#37009)) ;
#15189=EDGE_LOOP('',(#37010,#37011,#37012,#37013)) ;
#15190=EDGE_LOOP('',(#37014,#37015,#37016,#37017)) ;
#15191=EDGE_LOOP('',(#37018,#37019,#37020,#37021)) ;
#15192=EDGE_LOOP('',(#37022,#37023,#37024,#37025)) ;
#15193=EDGE_LOOP('',(#37026,#37027,#37028,#37029)) ;
#15194=EDGE_LOOP('',(#37030,#37031,#37032,#37033)) ;
#15195=EDGE_LOOP('',(#37034,#37035,#37036,#37037)) ;
#15196=EDGE_LOOP('',(#37038,#37039,#37040,#37041)) ;
#15197=EDGE_LOOP('',(#37042,#37043,#37044,#37045)) ;
#15198=EDGE_LOOP('',(#37046,#37047,#37048,#37049)) ;
#15199=EDGE_LOOP('',(#37050,#37051,#37052,#37053)) ;
#15200=EDGE_LOOP('',(#37054,#37055,#37056,#37057)) ;
#15201=EDGE_LOOP('',(#37058,#37059,#37060,#37061)) ;
#15202=EDGE_LOOP('',(#37062,#37063,#37064,#37065)) ;
#15203=EDGE_LOOP('',(#37066,#37067,#37068,#37069)) ;
#15204=EDGE_LOOP('',(#37070,#37071,#37072,#37073)) ;
#15205=EDGE_LOOP('',(#37074,#37075,#37076,#37077)) ;
#15206=EDGE_LOOP('',(#37078,#37079,#37080,#37081)) ;
#15207=EDGE_LOOP('',(#37082,#37083,#37084,#37085)) ;
#15208=EDGE_LOOP('',(#37086,#37087,#37088,#37089)) ;
#15209=EDGE_LOOP('',(#37090,#37091,#37092,#37093)) ;
#15210=EDGE_LOOP('',(#37094,#37095,#37096,#37097)) ;
#15211=EDGE_LOOP('',(#37098,#37099,#37100,#37101)) ;
#15212=EDGE_LOOP('',(#37102,#37103,#37104,#37105)) ;
#15213=EDGE_LOOP('',(#37106,#37107,#37108,#37109)) ;
#15214=EDGE_LOOP('',(#37110,#37111,#37112,#37113)) ;
#15215=EDGE_LOOP('',(#37114,#37115,#37116,#37117)) ;
#15216=EDGE_LOOP('',(#37118,#37119,#37120,#37121)) ;
#15217=EDGE_LOOP('',(#37122,#37123,#37124,#37125)) ;
#15218=EDGE_LOOP('',(#37126,#37127,#37128,#37129)) ;
#15219=EDGE_LOOP('',(#37130,#37131,#37132,#37133)) ;
#15220=EDGE_LOOP('',(#37134,#37135,#37136,#37137)) ;
#15221=EDGE_LOOP('',(#37138,#37139,#37140,#37141)) ;
#15222=EDGE_LOOP('',(#37142,#37143,#37144,#37145)) ;
#15223=EDGE_LOOP('',(#37146,#37147,#37148,#37149)) ;
#15224=EDGE_LOOP('',(#37150,#37151,#37152,#37153)) ;
#15225=EDGE_LOOP('',(#37154,#37155,#37156,#37157)) ;
#15226=EDGE_LOOP('',(#37158,#37159,#37160,#37161)) ;
#15227=EDGE_LOOP('',(#37162,#37163,#37164,#37165)) ;
#15228=EDGE_LOOP('',(#37166,#37167,#37168,#37169)) ;
#15229=EDGE_LOOP('',(#37170,#37171,#37172,#37173)) ;
#15230=EDGE_LOOP('',(#37174,#37175,#37176,#37177)) ;
#15231=EDGE_LOOP('',(#37178,#37179,#37180,#37181)) ;
#15232=EDGE_LOOP('',(#37182,#37183,#37184,#37185)) ;
#15233=EDGE_LOOP('',(#37186,#37187,#37188,#37189)) ;
#15234=EDGE_LOOP('',(#37190,#37191,#37192,#37193)) ;
#15235=EDGE_LOOP('',(#37194,#37195,#37196,#37197)) ;
#15236=EDGE_LOOP('',(#37198,#37199,#37200,#37201,#37202,#37203)) ;
#15237=EDGE_LOOP('',(#37204,#37205,#37206,#37207)) ;
#15238=EDGE_LOOP('',(#37208,#37209,#37210,#37211)) ;
#15239=EDGE_LOOP('',(#37212,#37213,#37214,#37215)) ;
#15240=EDGE_LOOP('',(#37216,#37217,#37218,#37219)) ;
#15241=EDGE_LOOP('',(#37220,#37221,#37222,#37223)) ;
#15242=EDGE_LOOP('',(#37224,#37225,#37226,#37227,#37228,#37229)) ;
#15243=EDGE_LOOP('',(#37230,#37231,#37232,#37233)) ;
#15244=EDGE_LOOP('',(#37234,#37235,#37236,#37237)) ;
#15245=EDGE_LOOP('',(#37238,#37239,#37240,#37241)) ;
#15246=EDGE_LOOP('',(#37242,#37243,#37244,#37245)) ;
#15247=EDGE_LOOP('',(#37246,#37247,#37248,#37249)) ;
#18278=CIRCLE('',#51736,0.100000000000016) ;
#18279=CIRCLE('',#51738,0.100000000000007) ;
#18280=CIRCLE('',#51739,0.100000000000016) ;
#18281=CIRCLE('',#51741,0.0999999999999979) ;
#18282=CIRCLE('',#51743,0.0999999999999973) ;
#18283=CIRCLE('',#51745,0.0999999999999973) ;
#18284=CIRCLE('',#51747,3.1) ;
#18285=CIRCLE('',#51748,0.1) ;
#18286=CIRCLE('',#51749,0.4) ;
#18287=CIRCLE('',#51750,0.4) ;
#18288=CIRCLE('',#51751,0.4) ;
#18289=CIRCLE('',#51752,2.4) ;
#18290=CIRCLE('',#51753,1.55266329058736) ;
#18291=CIRCLE('',#51754,1.55266329058736) ;
#18292=CIRCLE('',#51756,0.0999999999999979) ;
#18293=CIRCLE('',#51759,0.100000000000007) ;
#18294=CIRCLE('',#51761,2.4) ;
#18295=CIRCLE('',#51762,0.4) ;
#18296=CIRCLE('',#51763,0.4) ;
#18297=CIRCLE('',#51764,0.4) ;
#18298=CIRCLE('',#51765,0.1) ;
#18299=CIRCLE('',#51766,3.1) ;
#18300=CIRCLE('',#51767,1.45266329058736) ;
#18301=CIRCLE('',#51768,1.45266329058736) ;
#18302=CIRCLE('',#51770,0.1) ;
#18303=CIRCLE('',#51773,0.1) ;
#18304=CIRCLE('',#51777,0.0999999999999979) ;
#18305=CIRCLE('',#51778,0.0999999999999979) ;
#18306=CIRCLE('',#51779,0.5) ;
#18307=CIRCLE('',#51781,0.0999999999999979) ;
#18308=CIRCLE('',#51782,0.5) ;
#18309=CIRCLE('',#51783,0.0999999999999984) ;
#18310=CIRCLE('',#51787,0.0999999999999979) ;
#18311=CIRCLE('',#51789,0.0999999999999979) ;
#18312=CIRCLE('',#51791,0.0999999999999984) ;
#18313=CIRCLE('',#51792,0.0999999999999979) ;
#18314=CIRCLE('',#51793,0.5) ;
#18315=CIRCLE('',#51795,0.5) ;
#18316=CIRCLE('',#51796,0.0999999999999801) ;
#18317=CIRCLE('',#51801,0.0999999999999984) ;
#18318=CIRCLE('',#51802,0.0999999999999979) ;
#18319=CIRCLE('',#51803,0.5) ;
#18320=CIRCLE('',#51805,0.0999999999999979) ;
#18321=CIRCLE('',#51806,0.5) ;
#18322=CIRCLE('',#51809,0.0999999999999979) ;
#18323=CIRCLE('',#51812,0.100000000000012) ;
#18324=CIRCLE('',#51813,0.199999999999978) ;
#18325=CIRCLE('',#51819,0.199999999999996) ;
#18326=CIRCLE('',#51828,0.0999999999999979) ;
#18327=CIRCLE('',#51829,0.0999999999999801) ;
#18328=CIRCLE('',#51830,0.2) ;
#18329=CIRCLE('',#51831,0.2) ;
#18330=CIRCLE('',#51836,0.0999999999999979) ;
#18331=CIRCLE('',#51837,0.0999999999999979) ;
#18332=CIRCLE('',#51839,0.0999999999999979) ;
#18333=CIRCLE('',#51840,1.45266329058736) ;
#18334=CIRCLE('',#51842,0.0999999999999979) ;
#18335=CIRCLE('',#51844,1.45266329058736) ;
#18336=CIRCLE('',#51848,3.) ;
#18337=CIRCLE('',#51851,3.) ;
#18338=CIRCLE('',#51868,0.300000000000002) ;
#18339=CIRCLE('',#51869,1.19999999999999) ;
#18340=CIRCLE('',#51870,0.899999999999993) ;
#18341=CIRCLE('',#51872,0.300000000000002) ;
#18342=CIRCLE('',#51874,1.19999999999999) ;
#18343=CIRCLE('',#51875,0.899999999999993) ;
#18344=CIRCLE('',#51878,0.300000000000002) ;
#18345=CIRCLE('',#51879,1.19999999999999) ;
#18346=CIRCLE('',#51880,0.899999999999993) ;
#18347=CIRCLE('',#51882,0.300000000000002) ;
#18348=CIRCLE('',#51884,1.19999999999999) ;
#18349=CIRCLE('',#51885,0.899999999999993) ;
#18350=CIRCLE('',#51888,0.300000000000002) ;
#18351=CIRCLE('',#51889,1.19999999999999) ;
#18352=CIRCLE('',#51890,0.899999999999993) ;
#18353=CIRCLE('',#51892,0.300000000000002) ;
#18354=CIRCLE('',#51894,1.19999999999999) ;
#18355=CIRCLE('',#51895,0.899999999999993) ;
#18356=CIRCLE('',#51898,0.300000000000002) ;
#18357=CIRCLE('',#51899,1.19999999999999) ;
#18358=CIRCLE('',#51900,0.899999999999993) ;
#18359=CIRCLE('',#51902,0.300000000000002) ;
#18360=CIRCLE('',#51904,1.19999999999999) ;
#18361=CIRCLE('',#51905,0.899999999999993) ;
#18362=CIRCLE('',#51908,0.300000000000002) ;
#18363=CIRCLE('',#51909,1.19999999999999) ;
#18364=CIRCLE('',#51910,0.899999999999993) ;
#18365=CIRCLE('',#51912,0.300000000000002) ;
#18366=CIRCLE('',#51914,1.19999999999999) ;
#18367=CIRCLE('',#51915,0.899999999999993) ;
#18368=CIRCLE('',#51918,0.300000000000002) ;
#18369=CIRCLE('',#51919,1.19999999999999) ;
#18370=CIRCLE('',#51920,0.899999999999993) ;
#18371=CIRCLE('',#51922,0.300000000000002) ;
#18372=CIRCLE('',#51924,1.19999999999999) ;
#18373=CIRCLE('',#51925,0.899999999999993) ;
#18374=CIRCLE('',#51928,0.300000000000002) ;
#18375=CIRCLE('',#51929,1.19999999999999) ;
#18376=CIRCLE('',#51930,0.899999999999993) ;
#18377=CIRCLE('',#51932,0.300000000000002) ;
#18378=CIRCLE('',#51934,1.19999999999999) ;
#18379=CIRCLE('',#51935,0.899999999999993) ;
#18380=CIRCLE('',#51938,0.300000000000002) ;
#18381=CIRCLE('',#51939,1.19999999999999) ;
#18382=CIRCLE('',#51940,0.899999999999993) ;
#18383=CIRCLE('',#51942,0.300000000000002) ;
#18384=CIRCLE('',#51944,1.19999999999999) ;
#18385=CIRCLE('',#51945,0.899999999999993) ;
#21190=VERTEX_POINT('',#86613) ;
#21191=VERTEX_POINT('',#86614) ;
#21192=VERTEX_POINT('',#86625) ;
#21193=VERTEX_POINT('',#86627) ;
#21194=VERTEX_POINT('',#86631) ;
#21195=VERTEX_POINT('',#86633) ;
#21196=VERTEX_POINT('',#86635) ;
#21197=VERTEX_POINT('',#86639) ;
#21198=VERTEX_POINT('',#86640) ;
#21199=VERTEX_POINT('',#86651) ;
#21200=VERTEX_POINT('',#86660) ;
#21201=VERTEX_POINT('',#86662) ;
#21202=VERTEX_POINT('',#86664) ;
#21203=VERTEX_POINT('',#86666) ;
#21204=VERTEX_POINT('',#86668) ;
#21205=VERTEX_POINT('',#86670) ;
#21206=VERTEX_POINT('',#86672) ;
#21207=VERTEX_POINT('',#86674) ;
#21208=VERTEX_POINT('',#86676) ;
#21209=VERTEX_POINT('',#86678) ;
#21210=VERTEX_POINT('',#86680) ;
#21211=VERTEX_POINT('',#86682) ;
#21212=VERTEX_POINT('',#86684) ;
#21213=VERTEX_POINT('',#86686) ;
#21214=VERTEX_POINT('',#86688) ;
#21215=VERTEX_POINT('',#86690) ;
#21216=VERTEX_POINT('',#86692) ;
#21217=VERTEX_POINT('',#86694) ;
#21218=VERTEX_POINT('',#86696) ;
#21219=VERTEX_POINT('',#86698) ;
#21220=VERTEX_POINT('',#86700) ;
#21221=VERTEX_POINT('',#86702) ;
#21222=VERTEX_POINT('',#86704) ;
#21223=VERTEX_POINT('',#86707) ;
#21224=VERTEX_POINT('',#86708) ;
#21225=VERTEX_POINT('',#86710) ;
#21226=VERTEX_POINT('',#86712) ;
#21227=VERTEX_POINT('',#86715) ;
#21228=VERTEX_POINT('',#86716) ;
#21229=VERTEX_POINT('',#86727) ;
#21230=VERTEX_POINT('',#86729) ;
#21231=VERTEX_POINT('',#86740) ;
#21232=VERTEX_POINT('',#86742) ;
#21233=VERTEX_POINT('',#86753) ;
#21234=VERTEX_POINT('',#86755) ;
#21235=VERTEX_POINT('',#86767) ;
#21236=VERTEX_POINT('',#86768) ;
#21237=VERTEX_POINT('',#86770) ;
#21238=VERTEX_POINT('',#86781) ;
#21239=VERTEX_POINT('',#86783) ;
#21240=VERTEX_POINT('',#86794) ;
#21241=VERTEX_POINT('',#86796) ;
#21242=VERTEX_POINT('',#86807) ;
#21243=VERTEX_POINT('',#86819) ;
#21244=VERTEX_POINT('',#86820) ;
#21245=VERTEX_POINT('',#86822) ;
#21246=VERTEX_POINT('',#86833) ;
#21247=VERTEX_POINT('',#86835) ;
#21248=VERTEX_POINT('',#86846) ;
#21249=VERTEX_POINT('',#86848) ;
#21250=VERTEX_POINT('',#86859) ;
#21251=VERTEX_POINT('',#86871) ;
#21252=VERTEX_POINT('',#86872) ;
#21253=VERTEX_POINT('',#86874) ;
#21254=VERTEX_POINT('',#86885) ;
#21255=VERTEX_POINT('',#86887) ;
#21256=VERTEX_POINT('',#86898) ;
#21257=VERTEX_POINT('',#86900) ;
#21258=VERTEX_POINT('',#86911) ;
#21259=VERTEX_POINT('',#86924) ;
#21260=VERTEX_POINT('',#86928) ;
#21261=VERTEX_POINT('',#86932) ;
#21262=VERTEX_POINT('',#86936) ;
#21263=VERTEX_POINT('',#86938) ;
#21264=VERTEX_POINT('',#86940) ;
#21265=VERTEX_POINT('',#86942) ;
#21266=VERTEX_POINT('',#86944) ;
#21267=VERTEX_POINT('',#86946) ;
#21268=VERTEX_POINT('',#86948) ;
#21269=VERTEX_POINT('',#86950) ;
#21270=VERTEX_POINT('',#86952) ;
#21271=VERTEX_POINT('',#86954) ;
#21272=VERTEX_POINT('',#86956) ;
#21273=VERTEX_POINT('',#86958) ;
#21274=VERTEX_POINT('',#86960) ;
#21275=VERTEX_POINT('',#86962) ;
#21276=VERTEX_POINT('',#86964) ;
#21277=VERTEX_POINT('',#86966) ;
#21278=VERTEX_POINT('',#86968) ;
#21279=VERTEX_POINT('',#86970) ;
#21280=VERTEX_POINT('',#86972) ;
#21281=VERTEX_POINT('',#86974) ;
#21282=VERTEX_POINT('',#86976) ;
#21283=VERTEX_POINT('',#86978) ;
#21284=VERTEX_POINT('',#86981) ;
#21285=VERTEX_POINT('',#86982) ;
#21286=VERTEX_POINT('',#86984) ;
#21287=VERTEX_POINT('',#86986) ;
#21288=VERTEX_POINT('',#86989) ;
#21289=VERTEX_POINT('',#86990) ;
#21290=VERTEX_POINT('',#86992) ;
#21291=VERTEX_POINT('',#86994) ;
#21292=VERTEX_POINT('',#86998) ;
#21293=VERTEX_POINT('',#87000) ;
#21294=VERTEX_POINT('',#87004) ;
#21295=VERTEX_POINT('',#87006) ;
#21296=VERTEX_POINT('',#87013) ;
#21297=VERTEX_POINT('',#87015) ;
#21298=VERTEX_POINT('',#87019) ;
#21299=VERTEX_POINT('',#87021) ;
#21300=VERTEX_POINT('',#87028) ;
#21301=VERTEX_POINT('',#87030) ;
#21302=VERTEX_POINT('',#87036) ;
#21303=VERTEX_POINT('',#87040) ;
#21304=VERTEX_POINT('',#87042) ;
#21305=VERTEX_POINT('',#87046) ;
#21306=VERTEX_POINT('',#87056) ;
#21307=VERTEX_POINT('',#87061) ;
#21308=VERTEX_POINT('',#87067) ;
#21309=VERTEX_POINT('',#87071) ;
#21310=VERTEX_POINT('',#87101) ;
#21311=VERTEX_POINT('',#87102) ;
#21312=VERTEX_POINT('',#87104) ;
#21313=VERTEX_POINT('',#87107) ;
#21314=VERTEX_POINT('',#87111) ;
#21315=VERTEX_POINT('',#87113) ;
#21316=VERTEX_POINT('',#87141) ;
#21317=VERTEX_POINT('',#87144) ;
#21318=VERTEX_POINT('',#87148) ;
#21319=VERTEX_POINT('',#87150) ;
#21320=VERTEX_POINT('',#87156) ;
#21321=VERTEX_POINT('',#87168) ;
#21322=VERTEX_POINT('',#87187) ;
#21323=VERTEX_POINT('',#87189) ;
#21324=VERTEX_POINT('',#87193) ;
#21325=VERTEX_POINT('',#87197) ;
#21326=VERTEX_POINT('',#87208) ;
#21327=VERTEX_POINT('',#87215) ;
#21328=VERTEX_POINT('',#87222) ;
#21329=VERTEX_POINT('',#87224) ;
#21330=VERTEX_POINT('',#87244) ;
#21331=VERTEX_POINT('',#87253) ;
#21332=VERTEX_POINT('',#87263) ;
#21333=VERTEX_POINT('',#87264) ;
#21334=VERTEX_POINT('',#87269) ;
#21335=VERTEX_POINT('',#87270) ;
#21336=VERTEX_POINT('',#87279) ;
#21337=VERTEX_POINT('',#87280) ;
#21338=VERTEX_POINT('',#87285) ;
#21339=VERTEX_POINT('',#87286) ;
#21340=VERTEX_POINT('',#87295) ;
#21341=VERTEX_POINT('',#87296) ;
#21342=VERTEX_POINT('',#87301) ;
#21343=VERTEX_POINT('',#87302) ;
#21344=VERTEX_POINT('',#87311) ;
#21345=VERTEX_POINT('',#87312) ;
#21346=VERTEX_POINT('',#87317) ;
#21347=VERTEX_POINT('',#87318) ;
#21348=VERTEX_POINT('',#87327) ;
#21349=VERTEX_POINT('',#87328) ;
#21350=VERTEX_POINT('',#87333) ;
#21351=VERTEX_POINT('',#87334) ;
#21352=VERTEX_POINT('',#87343) ;
#21353=VERTEX_POINT('',#87344) ;
#21354=VERTEX_POINT('',#87349) ;
#21355=VERTEX_POINT('',#87350) ;
#21356=VERTEX_POINT('',#87359) ;
#21357=VERTEX_POINT('',#87360) ;
#21358=VERTEX_POINT('',#87365) ;
#21359=VERTEX_POINT('',#87366) ;
#21360=VERTEX_POINT('',#87375) ;
#21361=VERTEX_POINT('',#87376) ;
#21362=VERTEX_POINT('',#87381) ;
#21363=VERTEX_POINT('',#87382) ;
#21364=VERTEX_POINT('',#87411) ;
#21365=VERTEX_POINT('',#87412) ;
#21366=VERTEX_POINT('',#87414) ;
#21367=VERTEX_POINT('',#87416) ;
#26611=EDGE_CURVE('',#21190,#21191,#1127,.T.) ;
#26612=EDGE_CURVE('',#21191,#21192,#4105,.T.) ;
#26613=EDGE_CURVE('',#21192,#21193,#18278,.T.) ;
#26614=EDGE_CURVE('',#21193,#21190,#4106,.T.) ;
#26615=EDGE_CURVE('',#21194,#21192,#18279,.T.) ;
#26616=EDGE_CURVE('',#21192,#21195,#4107,.T.) ;
#26617=EDGE_CURVE('',#21195,#21196,#18280,.T.) ;
#26618=EDGE_CURVE('',#21196,#21194,#4108,.T.) ;
#26619=EDGE_CURVE('',#21197,#21198,#1128,.T.) ;
#26620=EDGE_CURVE('',#21198,#21199,#4109,.T.) ;
#26621=EDGE_CURVE('',#21199,#21195,#18281,.T.) ;
#26622=EDGE_CURVE('',#21195,#21197,#4110,.T.) ;
#26623=EDGE_CURVE('',#21199,#21196,#18282,.T.) ;
#26624=EDGE_CURVE('',#21194,#21193,#18283,.T.) ;
#26625=EDGE_CURVE('',#21200,#21193,#4111,.T.) ;
#26626=EDGE_CURVE('',#21201,#21200,#18284,.T.) ;
#26627=EDGE_CURVE('',#21202,#21201,#4112,.T.) ;
#26628=EDGE_CURVE('',#21203,#21202,#4113,.T.) ;
#26629=EDGE_CURVE('',#21204,#21203,#4114,.T.) ;
#26630=EDGE_CURVE('',#21205,#21204,#4115,.T.) ;
#26631=EDGE_CURVE('',#21206,#21205,#4116,.T.) ;
#26632=EDGE_CURVE('',#21207,#21206,#18285,.T.) ;
#26633=EDGE_CURVE('',#21208,#21207,#4117,.T.) ;
#26634=EDGE_CURVE('',#21209,#21208,#18286,.T.) ;
#26635=EDGE_CURVE('',#21210,#21209,#4118,.T.) ;
#26636=EDGE_CURVE('',#21211,#21210,#18287,.T.) ;
#26637=EDGE_CURVE('',#21212,#21211,#4119,.T.) ;
#26638=EDGE_CURVE('',#21213,#21212,#18288,.T.) ;
#26639=EDGE_CURVE('',#21214,#21213,#4120,.T.) ;
#26640=EDGE_CURVE('',#21215,#21214,#4121,.T.) ;
#26641=EDGE_CURVE('',#21216,#21215,#4122,.T.) ;
#26642=EDGE_CURVE('',#21217,#21216,#4123,.T.) ;
#26643=EDGE_CURVE('',#21218,#21217,#4124,.T.) ;
#26644=EDGE_CURVE('',#21219,#21218,#4125,.T.) ;
#26645=EDGE_CURVE('',#21220,#21219,#4126,.T.) ;
#26646=EDGE_CURVE('',#21221,#21220,#4127,.T.) ;
#26647=EDGE_CURVE('',#21221,#21222,#4128,.T.) ;
#26648=EDGE_CURVE('',#21222,#21190,#18289,.T.) ;
#26649=EDGE_CURVE('',#21223,#21224,#4129,.T.) ;
#26650=EDGE_CURVE('',#21225,#21223,#18290,.T.) ;
#26651=EDGE_CURVE('',#21226,#21225,#4130,.T.) ;
#26652=EDGE_CURVE('',#21224,#21226,#18291,.T.) ;
#26653=EDGE_CURVE('',#21227,#21228,#1129,.F.) ;
#26654=EDGE_CURVE('',#21229,#21227,#4131,.T.) ;
#26655=EDGE_CURVE('',#21230,#21229,#1130,.F.) ;
#26656=EDGE_CURVE('',#21231,#21230,#4132,.T.) ;
#26657=EDGE_CURVE('',#21232,#21231,#1131,.F.) ;
#26658=EDGE_CURVE('',#21233,#21232,#4133,.T.) ;
#26659=EDGE_CURVE('',#21234,#21233,#1132,.F.) ;
#26660=EDGE_CURVE('',#21228,#21234,#4134,.T.) ;
#26661=EDGE_CURVE('',#21235,#21236,#4135,.T.) ;
#26662=EDGE_CURVE('',#21237,#21236,#1133,.F.) ;
#26663=EDGE_CURVE('',#21237,#21238,#4136,.T.) ;
#26664=EDGE_CURVE('',#21239,#21238,#1134,.F.) ;
#26665=EDGE_CURVE('',#21239,#21240,#4137,.T.) ;
#26666=EDGE_CURVE('',#21241,#21240,#1135,.F.) ;
#26667=EDGE_CURVE('',#21241,#21242,#4138,.T.) ;
#26668=EDGE_CURVE('',#21235,#21242,#1136,.F.) ;
#26669=EDGE_CURVE('',#21243,#21244,#4139,.T.) ;
#26670=EDGE_CURVE('',#21245,#21244,#1137,.F.) ;
#26671=EDGE_CURVE('',#21245,#21246,#4140,.T.) ;
#26672=EDGE_CURVE('',#21247,#21246,#1138,.F.) ;
#26673=EDGE_CURVE('',#21247,#21248,#4141,.T.) ;
#26674=EDGE_CURVE('',#21249,#21248,#1139,.F.) ;
#26675=EDGE_CURVE('',#21249,#21250,#4142,.T.) ;
#26676=EDGE_CURVE('',#21243,#21250,#1140,.F.) ;
#26677=EDGE_CURVE('',#21251,#21252,#4143,.T.) ;
#26678=EDGE_CURVE('',#21253,#21252,#1141,.F.) ;
#26679=EDGE_CURVE('',#21253,#21254,#4144,.T.) ;
#26680=EDGE_CURVE('',#21255,#21254,#1142,.F.) ;
#26681=EDGE_CURVE('',#21255,#21256,#4145,.T.) ;
#26682=EDGE_CURVE('',#21257,#21256,#1143,.F.) ;
#26683=EDGE_CURVE('',#21257,#21258,#4146,.T.) ;
#26684=EDGE_CURVE('',#21251,#21258,#1144,.F.) ;
#26685=EDGE_CURVE('',#21194,#21259,#4147,.T.) ;
#26686=EDGE_CURVE('',#21200,#21259,#18292,.T.) ;
#26687=EDGE_CURVE('',#21260,#21196,#4148,.T.) ;
#26688=EDGE_CURVE('',#21259,#21260,#4149,.T.) ;
#26689=EDGE_CURVE('',#21199,#21261,#4150,.T.) ;
#26690=EDGE_CURVE('',#21260,#21261,#18293,.T.) ;
#26691=EDGE_CURVE('',#21198,#21262,#18294,.T.) ;
#26692=EDGE_CURVE('',#21262,#21263,#4151,.T.) ;
#26693=EDGE_CURVE('',#21263,#21264,#4152,.T.) ;
#26694=EDGE_CURVE('',#21264,#21265,#4153,.T.) ;
#26695=EDGE_CURVE('',#21265,#21266,#4154,.T.) ;
#26696=EDGE_CURVE('',#21266,#21267,#4155,.T.) ;
#26697=EDGE_CURVE('',#21267,#21268,#4156,.T.) ;
#26698=EDGE_CURVE('',#21268,#21269,#4157,.T.) ;
#26699=EDGE_CURVE('',#21270,#21269,#4158,.T.) ;
#26700=EDGE_CURVE('',#21271,#21270,#4159,.T.) ;
#26701=EDGE_CURVE('',#21272,#21271,#18295,.T.) ;
#26702=EDGE_CURVE('',#21273,#21272,#4160,.T.) ;
#26703=EDGE_CURVE('',#21274,#21273,#18296,.T.) ;
#26704=EDGE_CURVE('',#21275,#21274,#4161,.T.) ;
#26705=EDGE_CURVE('',#21276,#21275,#18297,.T.) ;
#26706=EDGE_CURVE('',#21277,#21276,#4162,.T.) ;
#26707=EDGE_CURVE('',#21278,#21277,#18298,.T.) ;
#26708=EDGE_CURVE('',#21279,#21278,#4163,.T.) ;
#26709=EDGE_CURVE('',#21280,#21279,#4164,.T.) ;
#26710=EDGE_CURVE('',#21281,#21280,#4165,.T.) ;
#26711=EDGE_CURVE('',#21281,#21282,#4166,.T.) ;
#26712=EDGE_CURVE('',#21282,#21283,#4167,.T.) ;
#26713=EDGE_CURVE('',#21261,#21283,#18299,.T.) ;
#26714=EDGE_CURVE('',#21284,#21285,#18300,.T.) ;
#26715=EDGE_CURVE('',#21285,#21286,#4168,.T.) ;
#26716=EDGE_CURVE('',#21286,#21287,#18301,.T.) ;
#26717=EDGE_CURVE('',#21287,#21284,#4169,.T.) ;
#26718=EDGE_CURVE('',#21288,#21289,#4170,.T.) ;
#26719=EDGE_CURVE('',#21289,#21290,#4171,.T.) ;
#26720=EDGE_CURVE('',#21290,#21291,#4172,.T.) ;
#26721=EDGE_CURVE('',#21291,#21288,#4173,.T.) ;
#26722=EDGE_CURVE('',#21269,#21292,#18302,.T.) ;
#26723=EDGE_CURVE('',#21292,#21293,#4174,.T.) ;
#26724=EDGE_CURVE('',#21293,#21270,#269,.F.) ;
#26725=EDGE_CURVE('',#21294,#21215,#18303,.T.) ;
#26726=EDGE_CURVE('',#21214,#21295,#270,.F.) ;
#26727=EDGE_CURVE('',#21295,#21294,#4175,.T.) ;
#26728=EDGE_CURVE('',#21294,#21292,#4176,.T.) ;
#26729=EDGE_CURVE('',#21295,#21293,#4177,.T.) ;
#26730=EDGE_CURVE('',#21296,#21274,#18304,.T.) ;
#26731=EDGE_CURVE('',#21273,#21297,#18305,.T.) ;
#26732=EDGE_CURVE('',#21297,#21296,#18306,.T.) ;
#26733=EDGE_CURVE('',#21210,#21298,#18307,.T.) ;
#26734=EDGE_CURVE('',#21298,#21299,#18308,.T.) ;
#26735=EDGE_CURVE('',#21299,#21211,#18309,.T.) ;
#26736=EDGE_CURVE('',#21298,#21296,#4178,.T.) ;
#26737=EDGE_CURVE('',#21297,#21299,#4179,.T.) ;
#26738=EDGE_CURVE('',#21300,#21298,#4180,.T.) ;
#26739=EDGE_CURVE('',#21301,#21300,#4181,.T.) ;
#26740=EDGE_CURVE('',#21296,#21301,#4182,.T.) ;
#26741=EDGE_CURVE('',#21300,#21209,#18310,.T.) ;
#26742=EDGE_CURVE('',#21299,#21302,#4183,.T.) ;
#26743=EDGE_CURVE('',#21212,#21302,#18311,.T.) ;
#26744=EDGE_CURVE('',#21303,#21272,#18312,.T.) ;
#26745=EDGE_CURVE('',#21271,#21304,#18313,.T.) ;
#26746=EDGE_CURVE('',#21304,#21303,#18314,.T.) ;
#26747=EDGE_CURVE('',#21302,#21305,#18315,.T.) ;
#26748=EDGE_CURVE('',#21305,#21213,#18316,.T.) ;
#26749=EDGE_CURVE('',#21302,#21303,#4184,.T.) ;
#26750=EDGE_CURVE('',#21304,#21305,#4185,.T.) ;
#26751=EDGE_CURVE('',#21303,#21297,#4186,.T.) ;
#26752=EDGE_CURVE('',#21306,#21276,#18317,.T.) ;
#26753=EDGE_CURVE('',#21275,#21301,#18318,.T.) ;
#26754=EDGE_CURVE('',#21301,#21306,#18319,.T.) ;
#26755=EDGE_CURVE('',#21208,#21307,#18320,.T.) ;
#26756=EDGE_CURVE('',#21307,#21300,#18321,.T.) ;
#26757=EDGE_CURVE('',#21307,#21306,#4187,.T.) ;
#26758=EDGE_CURVE('',#21306,#21308,#4188,.T.) ;
#26759=EDGE_CURVE('',#21277,#21308,#18322,.T.) ;
#26760=EDGE_CURVE('',#21309,#21307,#4189,.T.) ;
#26761=EDGE_CURVE('',#21308,#21309,#4190,.T.) ;
#26762=EDGE_CURVE('',#21309,#21207,#18323,.T.) ;
#26763=EDGE_CURVE('',#21310,#21311,#18324,.T.) ;
#26764=EDGE_CURVE('',#21311,#21312,#271,.T.) ;
#26765=EDGE_CURVE('',#21312,#21205,#272,.T.) ;
#26766=EDGE_CURVE('',#21205,#21313,#273,.T.) ;
#26767=EDGE_CURVE('',#21313,#21310,#274,.T.) ;
#26768=EDGE_CURVE('',#21310,#21314,#4191,.T.) ;
#26769=EDGE_CURVE('',#21314,#21315,#18325,.T.) ;
#26770=EDGE_CURVE('',#21315,#21311,#4192,.T.) ;
#26771=EDGE_CURVE('',#21314,#21316,#275,.T.) ;
#26772=EDGE_CURVE('',#21316,#21279,#276,.T.) ;
#26773=EDGE_CURVE('',#21279,#21317,#277,.T.) ;
#26774=EDGE_CURVE('',#21317,#21315,#278,.T.) ;
#26775=EDGE_CURVE('',#21318,#21310,#4193,.T.) ;
#26776=EDGE_CURVE('',#21318,#21319,#4194,.T.) ;
#26777=EDGE_CURVE('',#21314,#21319,#4195,.T.) ;
#26778=EDGE_CURVE('',#21204,#21318,#279,.T.) ;
#26779=EDGE_CURVE('',#21311,#21320,#4196,.T.) ;
#26780=EDGE_CURVE('',#21206,#21320,#18326,.T.) ;
#26781=EDGE_CURVE('',#21321,#21278,#18327,.T.) ;
#26782=EDGE_CURVE('',#21308,#21321,#18328,.T.) ;
#26783=EDGE_CURVE('',#21320,#21309,#18329,.T.) ;
#26784=EDGE_CURVE('',#21320,#21321,#4197,.T.) ;
#26785=EDGE_CURVE('',#21321,#21315,#4198,.T.) ;
#26786=EDGE_CURVE('',#21322,#21223,#18330,.T.) ;
#26787=EDGE_CURVE('',#21224,#21323,#18331,.T.) ;
#26788=EDGE_CURVE('',#21323,#21322,#4199,.T.) ;
#26789=EDGE_CURVE('',#21226,#21324,#18332,.T.) ;
#26790=EDGE_CURVE('',#21324,#21323,#18333,.T.) ;
#26791=EDGE_CURVE('',#21225,#21325,#18334,.T.) ;
#26792=EDGE_CURVE('',#21325,#21324,#4200,.T.) ;
#26793=EDGE_CURVE('',#21322,#21325,#18335,.T.) ;
#26794=EDGE_CURVE('',#21322,#21285,#4201,.T.) ;
#26795=EDGE_CURVE('',#21325,#21284,#4202,.T.) ;
#26796=EDGE_CURVE('',#21323,#21286,#4203,.T.) ;
#26797=EDGE_CURVE('',#21326,#21201,#1145,.T.) ;
#26798=EDGE_CURVE('',#21259,#21327,#18336,.T.) ;
#26799=EDGE_CURVE('',#21327,#21326,#1146,.T.) ;
#26800=EDGE_CURVE('',#21327,#21328,#4204,.T.) ;
#26801=EDGE_CURVE('',#21329,#21328,#1147,.T.) ;
#26802=EDGE_CURVE('',#21326,#21329,#4205,.T.) ;
#26803=EDGE_CURVE('',#21328,#21260,#18337,.T.) ;
#26804=EDGE_CURVE('',#21191,#21197,#4206,.T.) ;
#26805=EDGE_CURVE('',#21283,#21329,#1148,.T.) ;
#26806=EDGE_CURVE('',#21202,#21282,#4207,.T.) ;
#26807=EDGE_CURVE('',#21319,#21330,#4208,.T.) ;
#26808=EDGE_CURVE('',#21330,#21281,#280,.T.) ;
#26809=EDGE_CURVE('',#21280,#21319,#281,.T.) ;
#26810=EDGE_CURVE('',#21293,#21304,#4209,.T.) ;
#26811=EDGE_CURVE('',#21331,#21330,#4210,.T.) ;
#26812=EDGE_CURVE('',#21203,#21331,#282,.T.) ;
#26813=EDGE_CURVE('',#21331,#21318,#4211,.T.) ;
#26814=EDGE_CURVE('',#21305,#21295,#4212,.T.) ;
#26815=EDGE_CURVE('',#21332,#21333,#18338,.T.) ;
#26816=EDGE_CURVE('',#21333,#21255,#18339,.T.) ;
#26817=EDGE_CURVE('',#21254,#21332,#18340,.T.) ;
#26818=EDGE_CURVE('',#21334,#21335,#18341,.T.) ;
#26819=EDGE_CURVE('',#21335,#21333,#4213,.T.) ;
#26820=EDGE_CURVE('',#21332,#21334,#4214,.T.) ;
#26821=EDGE_CURVE('',#21252,#21335,#18342,.T.) ;
#26822=EDGE_CURVE('',#21334,#21253,#18343,.T.) ;
#26823=EDGE_CURVE('',#21336,#21337,#18344,.T.) ;
#26824=EDGE_CURVE('',#21337,#21251,#18345,.T.) ;
#26825=EDGE_CURVE('',#21258,#21336,#18346,.T.) ;
#26826=EDGE_CURVE('',#21338,#21339,#18347,.T.) ;
#26827=EDGE_CURVE('',#21339,#21337,#4215,.T.) ;
#26828=EDGE_CURVE('',#21336,#21338,#4216,.T.) ;
#26829=EDGE_CURVE('',#21256,#21339,#18348,.T.) ;
#26830=EDGE_CURVE('',#21338,#21257,#18349,.T.) ;
#26831=EDGE_CURVE('',#21340,#21341,#18350,.T.) ;
#26832=EDGE_CURVE('',#21341,#21235,#18351,.T.) ;
#26833=EDGE_CURVE('',#21242,#21340,#18352,.T.) ;
#26834=EDGE_CURVE('',#21342,#21343,#18353,.T.) ;
#26835=EDGE_CURVE('',#21343,#21341,#4217,.T.) ;
#26836=EDGE_CURVE('',#21340,#21342,#4218,.T.) ;
#26837=EDGE_CURVE('',#21240,#21343,#18354,.T.) ;
#26838=EDGE_CURVE('',#21342,#21241,#18355,.T.) ;
#26839=EDGE_CURVE('',#21344,#21345,#18356,.T.) ;
#26840=EDGE_CURVE('',#21345,#21239,#18357,.T.) ;
#26841=EDGE_CURVE('',#21238,#21344,#18358,.T.) ;
#26842=EDGE_CURVE('',#21346,#21347,#18359,.T.) ;
#26843=EDGE_CURVE('',#21347,#21345,#4219,.T.) ;
#26844=EDGE_CURVE('',#21344,#21346,#4220,.T.) ;
#26845=EDGE_CURVE('',#21236,#21347,#18360,.T.) ;
#26846=EDGE_CURVE('',#21346,#21237,#18361,.T.) ;
#26847=EDGE_CURVE('',#21348,#21349,#18362,.T.) ;
#26848=EDGE_CURVE('',#21349,#21243,#18363,.T.) ;
#26849=EDGE_CURVE('',#21250,#21348,#18364,.T.) ;
#26850=EDGE_CURVE('',#21350,#21351,#18365,.T.) ;
#26851=EDGE_CURVE('',#21351,#21349,#4221,.T.) ;
#26852=EDGE_CURVE('',#21348,#21350,#4222,.T.) ;
#26853=EDGE_CURVE('',#21248,#21351,#18366,.T.) ;
#26854=EDGE_CURVE('',#21350,#21249,#18367,.T.) ;
#26855=EDGE_CURVE('',#21352,#21353,#18368,.T.) ;
#26856=EDGE_CURVE('',#21353,#21247,#18369,.T.) ;
#26857=EDGE_CURVE('',#21246,#21352,#18370,.T.) ;
#26858=EDGE_CURVE('',#21354,#21355,#18371,.T.) ;
#26859=EDGE_CURVE('',#21355,#21353,#4223,.T.) ;
#26860=EDGE_CURVE('',#21352,#21354,#4224,.T.) ;
#26861=EDGE_CURVE('',#21244,#21355,#18372,.T.) ;
#26862=EDGE_CURVE('',#21354,#21245,#18373,.T.) ;
#26863=EDGE_CURVE('',#21356,#21357,#18374,.T.) ;
#26864=EDGE_CURVE('',#21357,#21227,#18375,.T.) ;
#26865=EDGE_CURVE('',#21228,#21356,#18376,.T.) ;
#26866=EDGE_CURVE('',#21358,#21359,#18377,.T.) ;
#26867=EDGE_CURVE('',#21359,#21357,#4225,.T.) ;
#26868=EDGE_CURVE('',#21356,#21358,#4226,.T.) ;
#26869=EDGE_CURVE('',#21233,#21359,#18378,.T.) ;
#26870=EDGE_CURVE('',#21358,#21234,#18379,.T.) ;
#26871=EDGE_CURVE('',#21360,#21361,#18380,.T.) ;
#26872=EDGE_CURVE('',#21361,#21232,#18381,.T.) ;
#26873=EDGE_CURVE('',#21231,#21360,#18382,.T.) ;
#26874=EDGE_CURVE('',#21362,#21363,#18383,.T.) ;
#26875=EDGE_CURVE('',#21363,#21361,#4227,.T.) ;
#26876=EDGE_CURVE('',#21360,#21362,#4228,.T.) ;
#26877=EDGE_CURVE('',#21229,#21363,#18384,.T.) ;
#26878=EDGE_CURVE('',#21362,#21230,#18385,.T.) ;
#26879=EDGE_CURVE('',#21361,#21359,#4229,.T.) ;
#26880=EDGE_CURVE('',#21357,#21363,#4230,.T.) ;
#26881=EDGE_CURVE('',#21353,#21351,#4231,.T.) ;
#26882=EDGE_CURVE('',#21349,#21355,#4232,.T.) ;
#26883=EDGE_CURVE('',#21341,#21347,#4233,.T.) ;
#26884=EDGE_CURVE('',#21345,#21343,#4234,.T.) ;
#26885=EDGE_CURVE('',#21333,#21339,#4235,.T.) ;
#26886=EDGE_CURVE('',#21337,#21335,#4236,.T.) ;
#26887=EDGE_CURVE('',#21364,#21365,#4237,.T.) ;
#26888=EDGE_CURVE('',#21366,#21364,#4238,.T.) ;
#26889=EDGE_CURVE('',#21367,#21366,#4239,.T.) ;
#26890=EDGE_CURVE('',#21365,#21367,#4240,.T.) ;
#26891=EDGE_CURVE('',#21367,#21290,#4241,.T.) ;
#26892=EDGE_CURVE('',#21365,#21289,#4242,.T.) ;
#26893=EDGE_CURVE('',#21366,#21291,#4243,.T.) ;
#26894=EDGE_CURVE('',#21262,#21222,#4244,.T.) ;
#26895=EDGE_CURVE('',#21221,#21263,#4245,.T.) ;
#26896=EDGE_CURVE('',#21324,#21287,#4246,.T.) ;
#26897=EDGE_CURVE('',#21364,#21288,#4247,.T.) ;
#26898=EDGE_CURVE('',#21216,#21268,#4248,.T.) ;
#26899=EDGE_CURVE('',#21217,#21267,#4249,.T.) ;
#26900=EDGE_CURVE('',#21218,#21266,#4250,.T.) ;
#26901=EDGE_CURVE('',#21219,#21265,#4251,.T.) ;
#26902=EDGE_CURVE('',#21220,#21264,#4252,.T.) ;
#36666=ORIENTED_EDGE('',*,*,#26611,.T.) ;
#36667=ORIENTED_EDGE('',*,*,#26612,.T.) ;
#36668=ORIENTED_EDGE('',*,*,#26613,.T.) ;
#36669=ORIENTED_EDGE('',*,*,#26614,.T.) ;
#36670=ORIENTED_EDGE('',*,*,#26615,.T.) ;
#36671=ORIENTED_EDGE('',*,*,#26616,.T.) ;
#36672=ORIENTED_EDGE('',*,*,#26617,.T.) ;
#36673=ORIENTED_EDGE('',*,*,#26618,.T.) ;
#36674=ORIENTED_EDGE('',*,*,#26619,.T.) ;
#36675=ORIENTED_EDGE('',*,*,#26620,.T.) ;
#36676=ORIENTED_EDGE('',*,*,#26621,.T.) ;
#36677=ORIENTED_EDGE('',*,*,#26622,.T.) ;
#36678=ORIENTED_EDGE('',*,*,#26621,.F.) ;
#36679=ORIENTED_EDGE('',*,*,#26623,.T.) ;
#36680=ORIENTED_EDGE('',*,*,#26617,.F.) ;
#36681=ORIENTED_EDGE('',*,*,#26615,.F.) ;
#36682=ORIENTED_EDGE('',*,*,#26624,.T.) ;
#36683=ORIENTED_EDGE('',*,*,#26613,.F.) ;
#36684=ORIENTED_EDGE('',*,*,#26614,.F.) ;
#36685=ORIENTED_EDGE('',*,*,#26625,.F.) ;
#36686=ORIENTED_EDGE('',*,*,#26626,.F.) ;
#36687=ORIENTED_EDGE('',*,*,#26627,.F.) ;
#36688=ORIENTED_EDGE('',*,*,#26628,.F.) ;
#36689=ORIENTED_EDGE('',*,*,#26629,.F.) ;
#36690=ORIENTED_EDGE('',*,*,#26630,.F.) ;
#36691=ORIENTED_EDGE('',*,*,#26631,.F.) ;
#36692=ORIENTED_EDGE('',*,*,#26632,.F.) ;
#36693=ORIENTED_EDGE('',*,*,#26633,.F.) ;
#36694=ORIENTED_EDGE('',*,*,#26634,.F.) ;
#36695=ORIENTED_EDGE('',*,*,#26635,.F.) ;
#36696=ORIENTED_EDGE('',*,*,#26636,.F.) ;
#36697=ORIENTED_EDGE('',*,*,#26637,.F.) ;
#36698=ORIENTED_EDGE('',*,*,#26638,.F.) ;
#36699=ORIENTED_EDGE('',*,*,#26639,.F.) ;
#36700=ORIENTED_EDGE('',*,*,#26640,.F.) ;
#36701=ORIENTED_EDGE('',*,*,#26641,.F.) ;
#36702=ORIENTED_EDGE('',*,*,#26642,.F.) ;
#36703=ORIENTED_EDGE('',*,*,#26643,.F.) ;
#36704=ORIENTED_EDGE('',*,*,#26644,.F.) ;
#36705=ORIENTED_EDGE('',*,*,#26645,.F.) ;
#36706=ORIENTED_EDGE('',*,*,#26646,.F.) ;
#36707=ORIENTED_EDGE('',*,*,#26647,.T.) ;
#36708=ORIENTED_EDGE('',*,*,#26648,.T.) ;
#36709=ORIENTED_EDGE('',*,*,#26649,.F.) ;
#36710=ORIENTED_EDGE('',*,*,#26650,.F.) ;
#36711=ORIENTED_EDGE('',*,*,#26651,.F.) ;
#36712=ORIENTED_EDGE('',*,*,#26652,.F.) ;
#36713=ORIENTED_EDGE('',*,*,#26653,.F.) ;
#36714=ORIENTED_EDGE('',*,*,#26654,.F.) ;
#36715=ORIENTED_EDGE('',*,*,#26655,.F.) ;
#36716=ORIENTED_EDGE('',*,*,#26656,.F.) ;
#36717=ORIENTED_EDGE('',*,*,#26657,.F.) ;
#36718=ORIENTED_EDGE('',*,*,#26658,.F.) ;
#36719=ORIENTED_EDGE('',*,*,#26659,.F.) ;
#36720=ORIENTED_EDGE('',*,*,#26660,.F.) ;
#36721=ORIENTED_EDGE('',*,*,#26661,.T.) ;
#36722=ORIENTED_EDGE('',*,*,#26662,.F.) ;
#36723=ORIENTED_EDGE('',*,*,#26663,.T.) ;
#36724=ORIENTED_EDGE('',*,*,#26664,.F.) ;
#36725=ORIENTED_EDGE('',*,*,#26665,.T.) ;
#36726=ORIENTED_EDGE('',*,*,#26666,.F.) ;
#36727=ORIENTED_EDGE('',*,*,#26667,.T.) ;
#36728=ORIENTED_EDGE('',*,*,#26668,.F.) ;
#36729=ORIENTED_EDGE('',*,*,#26669,.T.) ;
#36730=ORIENTED_EDGE('',*,*,#26670,.F.) ;
#36731=ORIENTED_EDGE('',*,*,#26671,.T.) ;
#36732=ORIENTED_EDGE('',*,*,#26672,.F.) ;
#36733=ORIENTED_EDGE('',*,*,#26673,.T.) ;
#36734=ORIENTED_EDGE('',*,*,#26674,.F.) ;
#36735=ORIENTED_EDGE('',*,*,#26675,.T.) ;
#36736=ORIENTED_EDGE('',*,*,#26676,.F.) ;
#36737=ORIENTED_EDGE('',*,*,#26677,.T.) ;
#36738=ORIENTED_EDGE('',*,*,#26678,.F.) ;
#36739=ORIENTED_EDGE('',*,*,#26679,.T.) ;
#36740=ORIENTED_EDGE('',*,*,#26680,.F.) ;
#36741=ORIENTED_EDGE('',*,*,#26681,.T.) ;
#36742=ORIENTED_EDGE('',*,*,#26682,.F.) ;
#36743=ORIENTED_EDGE('',*,*,#26683,.T.) ;
#36744=ORIENTED_EDGE('',*,*,#26684,.F.) ;
#36745=ORIENTED_EDGE('',*,*,#26624,.F.) ;
#36746=ORIENTED_EDGE('',*,*,#26685,.T.) ;
#36747=ORIENTED_EDGE('',*,*,#26686,.F.) ;
#36748=ORIENTED_EDGE('',*,*,#26625,.T.) ;
#36749=ORIENTED_EDGE('',*,*,#26618,.F.) ;
#36750=ORIENTED_EDGE('',*,*,#26687,.F.) ;
#36751=ORIENTED_EDGE('',*,*,#26688,.F.) ;
#36752=ORIENTED_EDGE('',*,*,#26685,.F.) ;
#36753=ORIENTED_EDGE('',*,*,#26623,.F.) ;
#36754=ORIENTED_EDGE('',*,*,#26689,.T.) ;
#36755=ORIENTED_EDGE('',*,*,#26690,.F.) ;
#36756=ORIENTED_EDGE('',*,*,#26687,.T.) ;
#36757=ORIENTED_EDGE('',*,*,#26620,.F.) ;
#36758=ORIENTED_EDGE('',*,*,#26691,.T.) ;
#36759=ORIENTED_EDGE('',*,*,#26692,.T.) ;
#36760=ORIENTED_EDGE('',*,*,#26693,.T.) ;
#36761=ORIENTED_EDGE('',*,*,#26694,.T.) ;
#36762=ORIENTED_EDGE('',*,*,#26695,.T.) ;
#36763=ORIENTED_EDGE('',*,*,#26696,.T.) ;
#36764=ORIENTED_EDGE('',*,*,#26697,.T.) ;
#36765=ORIENTED_EDGE('',*,*,#26698,.T.) ;
#36766=ORIENTED_EDGE('',*,*,#26699,.F.) ;
#36767=ORIENTED_EDGE('',*,*,#26700,.F.) ;
#36768=ORIENTED_EDGE('',*,*,#26701,.F.) ;
#36769=ORIENTED_EDGE('',*,*,#26702,.F.) ;
#36770=ORIENTED_EDGE('',*,*,#26703,.F.) ;
#36771=ORIENTED_EDGE('',*,*,#26704,.F.) ;
#36772=ORIENTED_EDGE('',*,*,#26705,.F.) ;
#36773=ORIENTED_EDGE('',*,*,#26706,.F.) ;
#36774=ORIENTED_EDGE('',*,*,#26707,.F.) ;
#36775=ORIENTED_EDGE('',*,*,#26708,.F.) ;
#36776=ORIENTED_EDGE('',*,*,#26709,.F.) ;
#36777=ORIENTED_EDGE('',*,*,#26710,.F.) ;
#36778=ORIENTED_EDGE('',*,*,#26711,.T.) ;
#36779=ORIENTED_EDGE('',*,*,#26712,.T.) ;
#36780=ORIENTED_EDGE('',*,*,#26713,.F.) ;
#36781=ORIENTED_EDGE('',*,*,#26689,.F.) ;
#36782=ORIENTED_EDGE('',*,*,#26714,.T.) ;
#36783=ORIENTED_EDGE('',*,*,#26715,.T.) ;
#36784=ORIENTED_EDGE('',*,*,#26716,.T.) ;
#36785=ORIENTED_EDGE('',*,*,#26717,.T.) ;
#36786=ORIENTED_EDGE('',*,*,#26718,.T.) ;
#36787=ORIENTED_EDGE('',*,*,#26719,.T.) ;
#36788=ORIENTED_EDGE('',*,*,#26720,.T.) ;
#36789=ORIENTED_EDGE('',*,*,#26721,.T.) ;
#36790=ORIENTED_EDGE('',*,*,#26722,.T.) ;
#36791=ORIENTED_EDGE('',*,*,#26723,.T.) ;
#36792=ORIENTED_EDGE('',*,*,#26724,.T.) ;
#36793=ORIENTED_EDGE('',*,*,#26699,.T.) ;
#36794=ORIENTED_EDGE('',*,*,#26725,.T.) ;
#36795=ORIENTED_EDGE('',*,*,#26640,.T.) ;
#36796=ORIENTED_EDGE('',*,*,#26726,.T.) ;
#36797=ORIENTED_EDGE('',*,*,#26727,.T.) ;
#36798=ORIENTED_EDGE('',*,*,#26723,.F.) ;
#36799=ORIENTED_EDGE('',*,*,#26728,.F.) ;
#36800=ORIENTED_EDGE('',*,*,#26727,.F.) ;
#36801=ORIENTED_EDGE('',*,*,#26729,.T.) ;
#36802=ORIENTED_EDGE('',*,*,#26730,.T.) ;
#36803=ORIENTED_EDGE('',*,*,#26703,.T.) ;
#36804=ORIENTED_EDGE('',*,*,#26731,.T.) ;
#36805=ORIENTED_EDGE('',*,*,#26732,.T.) ;
#36806=ORIENTED_EDGE('',*,*,#26733,.T.) ;
#36807=ORIENTED_EDGE('',*,*,#26734,.T.) ;
#36808=ORIENTED_EDGE('',*,*,#26735,.T.) ;
#36809=ORIENTED_EDGE('',*,*,#26636,.T.) ;
#36810=ORIENTED_EDGE('',*,*,#26734,.F.) ;
#36811=ORIENTED_EDGE('',*,*,#26736,.T.) ;
#36812=ORIENTED_EDGE('',*,*,#26732,.F.) ;
#36813=ORIENTED_EDGE('',*,*,#26737,.T.) ;
#36814=ORIENTED_EDGE('',*,*,#26736,.F.) ;
#36815=ORIENTED_EDGE('',*,*,#26738,.F.) ;
#36816=ORIENTED_EDGE('',*,*,#26739,.F.) ;
#36817=ORIENTED_EDGE('',*,*,#26740,.F.) ;
#36818=ORIENTED_EDGE('',*,*,#26733,.F.) ;
#36819=ORIENTED_EDGE('',*,*,#26635,.T.) ;
#36820=ORIENTED_EDGE('',*,*,#26741,.F.) ;
#36821=ORIENTED_EDGE('',*,*,#26738,.T.) ;
#36822=ORIENTED_EDGE('',*,*,#26735,.F.) ;
#36823=ORIENTED_EDGE('',*,*,#26742,.T.) ;
#36824=ORIENTED_EDGE('',*,*,#26743,.F.) ;
#36825=ORIENTED_EDGE('',*,*,#26637,.T.) ;
#36826=ORIENTED_EDGE('',*,*,#26744,.T.) ;
#36827=ORIENTED_EDGE('',*,*,#26701,.T.) ;
#36828=ORIENTED_EDGE('',*,*,#26745,.T.) ;
#36829=ORIENTED_EDGE('',*,*,#26746,.T.) ;
#36830=ORIENTED_EDGE('',*,*,#26743,.T.) ;
#36831=ORIENTED_EDGE('',*,*,#26747,.T.) ;
#36832=ORIENTED_EDGE('',*,*,#26748,.T.) ;
#36833=ORIENTED_EDGE('',*,*,#26638,.T.) ;
#36834=ORIENTED_EDGE('',*,*,#26747,.F.) ;
#36835=ORIENTED_EDGE('',*,*,#26749,.T.) ;
#36836=ORIENTED_EDGE('',*,*,#26746,.F.) ;
#36837=ORIENTED_EDGE('',*,*,#26750,.T.) ;
#36838=ORIENTED_EDGE('',*,*,#26731,.F.) ;
#36839=ORIENTED_EDGE('',*,*,#26702,.T.) ;
#36840=ORIENTED_EDGE('',*,*,#26744,.F.) ;
#36841=ORIENTED_EDGE('',*,*,#26751,.T.) ;
#36842=ORIENTED_EDGE('',*,*,#26737,.F.) ;
#36843=ORIENTED_EDGE('',*,*,#26751,.F.) ;
#36844=ORIENTED_EDGE('',*,*,#26749,.F.) ;
#36845=ORIENTED_EDGE('',*,*,#26742,.F.) ;
#36846=ORIENTED_EDGE('',*,*,#26752,.T.) ;
#36847=ORIENTED_EDGE('',*,*,#26705,.T.) ;
#36848=ORIENTED_EDGE('',*,*,#26753,.T.) ;
#36849=ORIENTED_EDGE('',*,*,#26754,.T.) ;
#36850=ORIENTED_EDGE('',*,*,#26755,.T.) ;
#36851=ORIENTED_EDGE('',*,*,#26756,.T.) ;
#36852=ORIENTED_EDGE('',*,*,#26741,.T.) ;
#36853=ORIENTED_EDGE('',*,*,#26634,.T.) ;
#36854=ORIENTED_EDGE('',*,*,#26756,.F.) ;
#36855=ORIENTED_EDGE('',*,*,#26757,.T.) ;
#36856=ORIENTED_EDGE('',*,*,#26754,.F.) ;
#36857=ORIENTED_EDGE('',*,*,#26739,.T.) ;
#36858=ORIENTED_EDGE('',*,*,#26752,.F.) ;
#36859=ORIENTED_EDGE('',*,*,#26758,.T.) ;
#36860=ORIENTED_EDGE('',*,*,#26759,.F.) ;
#36861=ORIENTED_EDGE('',*,*,#26706,.T.) ;
#36862=ORIENTED_EDGE('',*,*,#26757,.F.) ;
#36863=ORIENTED_EDGE('',*,*,#26760,.F.) ;
#36864=ORIENTED_EDGE('',*,*,#26761,.F.) ;
#36865=ORIENTED_EDGE('',*,*,#26758,.F.) ;
#36866=ORIENTED_EDGE('',*,*,#26755,.F.) ;
#36867=ORIENTED_EDGE('',*,*,#26633,.T.) ;
#36868=ORIENTED_EDGE('',*,*,#26762,.F.) ;
#36869=ORIENTED_EDGE('',*,*,#26760,.T.) ;
#36870=ORIENTED_EDGE('',*,*,#26763,.T.) ;
#36871=ORIENTED_EDGE('',*,*,#26764,.T.) ;
#36872=ORIENTED_EDGE('',*,*,#26765,.T.) ;
#36873=ORIENTED_EDGE('',*,*,#26766,.T.) ;
#36874=ORIENTED_EDGE('',*,*,#26767,.T.) ;
#36875=ORIENTED_EDGE('',*,*,#26763,.F.) ;
#36876=ORIENTED_EDGE('',*,*,#26768,.T.) ;
#36877=ORIENTED_EDGE('',*,*,#26769,.T.) ;
#36878=ORIENTED_EDGE('',*,*,#26770,.T.) ;
#36879=ORIENTED_EDGE('',*,*,#26769,.F.) ;
#36880=ORIENTED_EDGE('',*,*,#26771,.T.) ;
#36881=ORIENTED_EDGE('',*,*,#26772,.T.) ;
#36882=ORIENTED_EDGE('',*,*,#26773,.T.) ;
#36883=ORIENTED_EDGE('',*,*,#26774,.T.) ;
#36884=ORIENTED_EDGE('',*,*,#26768,.F.) ;
#36885=ORIENTED_EDGE('',*,*,#26775,.F.) ;
#36886=ORIENTED_EDGE('',*,*,#26776,.T.) ;
#36887=ORIENTED_EDGE('',*,*,#26777,.F.) ;
#36888=ORIENTED_EDGE('',*,*,#26766,.F.) ;
#36889=ORIENTED_EDGE('',*,*,#26630,.T.) ;
#36890=ORIENTED_EDGE('',*,*,#26778,.T.) ;
#36891=ORIENTED_EDGE('',*,*,#26775,.T.) ;
#36892=ORIENTED_EDGE('',*,*,#26767,.F.) ;
#36893=ORIENTED_EDGE('',*,*,#26764,.F.) ;
#36894=ORIENTED_EDGE('',*,*,#26779,.T.) ;
#36895=ORIENTED_EDGE('',*,*,#26780,.F.) ;
#36896=ORIENTED_EDGE('',*,*,#26631,.T.) ;
#36897=ORIENTED_EDGE('',*,*,#26765,.F.) ;
#36898=ORIENTED_EDGE('',*,*,#26781,.T.) ;
#36899=ORIENTED_EDGE('',*,*,#26707,.T.) ;
#36900=ORIENTED_EDGE('',*,*,#26759,.T.) ;
#36901=ORIENTED_EDGE('',*,*,#26782,.T.) ;
#36902=ORIENTED_EDGE('',*,*,#26780,.T.) ;
#36903=ORIENTED_EDGE('',*,*,#26783,.T.) ;
#36904=ORIENTED_EDGE('',*,*,#26762,.T.) ;
#36905=ORIENTED_EDGE('',*,*,#26632,.T.) ;
#36906=ORIENTED_EDGE('',*,*,#26783,.F.) ;
#36907=ORIENTED_EDGE('',*,*,#26784,.T.) ;
#36908=ORIENTED_EDGE('',*,*,#26782,.F.) ;
#36909=ORIENTED_EDGE('',*,*,#26761,.T.) ;
#36910=ORIENTED_EDGE('',*,*,#26773,.F.) ;
#36911=ORIENTED_EDGE('',*,*,#26708,.T.) ;
#36912=ORIENTED_EDGE('',*,*,#26781,.F.) ;
#36913=ORIENTED_EDGE('',*,*,#26785,.T.) ;
#36914=ORIENTED_EDGE('',*,*,#26774,.F.) ;
#36915=ORIENTED_EDGE('',*,*,#26770,.F.) ;
#36916=ORIENTED_EDGE('',*,*,#26785,.F.) ;
#36917=ORIENTED_EDGE('',*,*,#26784,.F.) ;
#36918=ORIENTED_EDGE('',*,*,#26779,.F.) ;
#36919=ORIENTED_EDGE('',*,*,#26786,.T.) ;
#36920=ORIENTED_EDGE('',*,*,#26649,.T.) ;
#36921=ORIENTED_EDGE('',*,*,#26787,.T.) ;
#36922=ORIENTED_EDGE('',*,*,#26788,.T.) ;
#36923=ORIENTED_EDGE('',*,*,#26789,.T.) ;
#36924=ORIENTED_EDGE('',*,*,#26790,.T.) ;
#36925=ORIENTED_EDGE('',*,*,#26787,.F.) ;
#36926=ORIENTED_EDGE('',*,*,#26652,.T.) ;
#36927=ORIENTED_EDGE('',*,*,#26791,.T.) ;
#36928=ORIENTED_EDGE('',*,*,#26792,.T.) ;
#36929=ORIENTED_EDGE('',*,*,#26789,.F.) ;
#36930=ORIENTED_EDGE('',*,*,#26651,.T.) ;
#36931=ORIENTED_EDGE('',*,*,#26786,.F.) ;
#36932=ORIENTED_EDGE('',*,*,#26793,.T.) ;
#36933=ORIENTED_EDGE('',*,*,#26791,.F.) ;
#36934=ORIENTED_EDGE('',*,*,#26650,.T.) ;
#36935=ORIENTED_EDGE('',*,*,#26793,.F.) ;
#36936=ORIENTED_EDGE('',*,*,#26794,.T.) ;
#36937=ORIENTED_EDGE('',*,*,#26714,.F.) ;
#36938=ORIENTED_EDGE('',*,*,#26795,.F.) ;
#36939=ORIENTED_EDGE('',*,*,#26788,.F.) ;
#36940=ORIENTED_EDGE('',*,*,#26796,.T.) ;
#36941=ORIENTED_EDGE('',*,*,#26715,.F.) ;
#36942=ORIENTED_EDGE('',*,*,#26794,.F.) ;
#36943=ORIENTED_EDGE('',*,*,#26797,.T.) ;
#36944=ORIENTED_EDGE('',*,*,#26626,.T.) ;
#36945=ORIENTED_EDGE('',*,*,#26686,.T.) ;
#36946=ORIENTED_EDGE('',*,*,#26798,.T.) ;
#36947=ORIENTED_EDGE('',*,*,#26799,.T.) ;
#36948=ORIENTED_EDGE('',*,*,#26799,.F.) ;
#36949=ORIENTED_EDGE('',*,*,#26800,.T.) ;
#36950=ORIENTED_EDGE('',*,*,#26801,.F.) ;
#36951=ORIENTED_EDGE('',*,*,#26802,.F.) ;
#36952=ORIENTED_EDGE('',*,*,#26798,.F.) ;
#36953=ORIENTED_EDGE('',*,*,#26688,.T.) ;
#36954=ORIENTED_EDGE('',*,*,#26803,.F.) ;
#36955=ORIENTED_EDGE('',*,*,#26800,.F.) ;
#36956=ORIENTED_EDGE('',*,*,#26612,.F.) ;
#36957=ORIENTED_EDGE('',*,*,#26804,.T.) ;
#36958=ORIENTED_EDGE('',*,*,#26622,.F.) ;
#36959=ORIENTED_EDGE('',*,*,#26616,.F.) ;
#36960=ORIENTED_EDGE('',*,*,#26801,.T.) ;
#36961=ORIENTED_EDGE('',*,*,#26803,.T.) ;
#36962=ORIENTED_EDGE('',*,*,#26690,.T.) ;
#36963=ORIENTED_EDGE('',*,*,#26713,.T.) ;
#36964=ORIENTED_EDGE('',*,*,#26805,.T.) ;
#36965=ORIENTED_EDGE('',*,*,#26797,.F.) ;
#36966=ORIENTED_EDGE('',*,*,#26802,.T.) ;
#36967=ORIENTED_EDGE('',*,*,#26805,.F.) ;
#36968=ORIENTED_EDGE('',*,*,#26712,.F.) ;
#36969=ORIENTED_EDGE('',*,*,#26806,.F.) ;
#36970=ORIENTED_EDGE('',*,*,#26627,.T.) ;
#36971=ORIENTED_EDGE('',*,*,#26807,.T.) ;
#36972=ORIENTED_EDGE('',*,*,#26808,.T.) ;
#36973=ORIENTED_EDGE('',*,*,#26710,.T.) ;
#36974=ORIENTED_EDGE('',*,*,#26809,.T.) ;
#36975=ORIENTED_EDGE('',*,*,#26771,.F.) ;
#36976=ORIENTED_EDGE('',*,*,#26777,.T.) ;
#36977=ORIENTED_EDGE('',*,*,#26809,.F.) ;
#36978=ORIENTED_EDGE('',*,*,#26709,.T.) ;
#36979=ORIENTED_EDGE('',*,*,#26772,.F.) ;
#36980=ORIENTED_EDGE('',*,*,#26730,.F.) ;
#36981=ORIENTED_EDGE('',*,*,#26740,.T.) ;
#36982=ORIENTED_EDGE('',*,*,#26753,.F.) ;
#36983=ORIENTED_EDGE('',*,*,#26704,.T.) ;
#36984=ORIENTED_EDGE('',*,*,#26745,.F.) ;
#36985=ORIENTED_EDGE('',*,*,#26700,.T.) ;
#36986=ORIENTED_EDGE('',*,*,#26724,.F.) ;
#36987=ORIENTED_EDGE('',*,*,#26810,.T.) ;
#36988=ORIENTED_EDGE('',*,*,#26808,.F.) ;
#36989=ORIENTED_EDGE('',*,*,#26811,.F.) ;
#36990=ORIENTED_EDGE('',*,*,#26812,.F.) ;
#36991=ORIENTED_EDGE('',*,*,#26628,.T.) ;
#36992=ORIENTED_EDGE('',*,*,#26806,.T.) ;
#36993=ORIENTED_EDGE('',*,*,#26711,.F.) ;
#36994=ORIENTED_EDGE('',*,*,#26807,.F.) ;
#36995=ORIENTED_EDGE('',*,*,#26776,.F.) ;
#36996=ORIENTED_EDGE('',*,*,#26813,.F.) ;
#36997=ORIENTED_EDGE('',*,*,#26811,.T.) ;
#36998=ORIENTED_EDGE('',*,*,#26750,.F.) ;
#36999=ORIENTED_EDGE('',*,*,#26810,.F.) ;
#37000=ORIENTED_EDGE('',*,*,#26729,.F.) ;
#37001=ORIENTED_EDGE('',*,*,#26814,.F.) ;
#37002=ORIENTED_EDGE('',*,*,#26748,.F.) ;
#37003=ORIENTED_EDGE('',*,*,#26814,.T.) ;
#37004=ORIENTED_EDGE('',*,*,#26726,.F.) ;
#37005=ORIENTED_EDGE('',*,*,#26639,.T.) ;
#37006=ORIENTED_EDGE('',*,*,#26629,.T.) ;
#37007=ORIENTED_EDGE('',*,*,#26812,.T.) ;
#37008=ORIENTED_EDGE('',*,*,#26813,.T.) ;
#37009=ORIENTED_EDGE('',*,*,#26778,.F.) ;
#37010=ORIENTED_EDGE('',*,*,#26815,.T.) ;
#37011=ORIENTED_EDGE('',*,*,#26816,.T.) ;
#37012=ORIENTED_EDGE('',*,*,#26680,.T.) ;
#37013=ORIENTED_EDGE('',*,*,#26817,.T.) ;
#37014=ORIENTED_EDGE('',*,*,#26818,.T.) ;
#37015=ORIENTED_EDGE('',*,*,#26819,.T.) ;
#37016=ORIENTED_EDGE('',*,*,#26815,.F.) ;
#37017=ORIENTED_EDGE('',*,*,#26820,.T.) ;
#37018=ORIENTED_EDGE('',*,*,#26678,.T.) ;
#37019=ORIENTED_EDGE('',*,*,#26821,.T.) ;
#37020=ORIENTED_EDGE('',*,*,#26818,.F.) ;
#37021=ORIENTED_EDGE('',*,*,#26822,.T.) ;
#37022=ORIENTED_EDGE('',*,*,#26822,.F.) ;
#37023=ORIENTED_EDGE('',*,*,#26820,.F.) ;
#37024=ORIENTED_EDGE('',*,*,#26817,.F.) ;
#37025=ORIENTED_EDGE('',*,*,#26679,.F.) ;
#37026=ORIENTED_EDGE('',*,*,#26823,.T.) ;
#37027=ORIENTED_EDGE('',*,*,#26824,.T.) ;
#37028=ORIENTED_EDGE('',*,*,#26684,.T.) ;
#37029=ORIENTED_EDGE('',*,*,#26825,.T.) ;
#37030=ORIENTED_EDGE('',*,*,#26826,.T.) ;
#37031=ORIENTED_EDGE('',*,*,#26827,.T.) ;
#37032=ORIENTED_EDGE('',*,*,#26823,.F.) ;
#37033=ORIENTED_EDGE('',*,*,#26828,.T.) ;
#37034=ORIENTED_EDGE('',*,*,#26682,.T.) ;
#37035=ORIENTED_EDGE('',*,*,#26829,.T.) ;
#37036=ORIENTED_EDGE('',*,*,#26826,.F.) ;
#37037=ORIENTED_EDGE('',*,*,#26830,.T.) ;
#37038=ORIENTED_EDGE('',*,*,#26830,.F.) ;
#37039=ORIENTED_EDGE('',*,*,#26828,.F.) ;
#37040=ORIENTED_EDGE('',*,*,#26825,.F.) ;
#37041=ORIENTED_EDGE('',*,*,#26683,.F.) ;
#37042=ORIENTED_EDGE('',*,*,#26831,.T.) ;
#37043=ORIENTED_EDGE('',*,*,#26832,.T.) ;
#37044=ORIENTED_EDGE('',*,*,#26668,.T.) ;
#37045=ORIENTED_EDGE('',*,*,#26833,.T.) ;
#37046=ORIENTED_EDGE('',*,*,#26834,.T.) ;
#37047=ORIENTED_EDGE('',*,*,#26835,.T.) ;
#37048=ORIENTED_EDGE('',*,*,#26831,.F.) ;
#37049=ORIENTED_EDGE('',*,*,#26836,.T.) ;
#37050=ORIENTED_EDGE('',*,*,#26666,.T.) ;
#37051=ORIENTED_EDGE('',*,*,#26837,.T.) ;
#37052=ORIENTED_EDGE('',*,*,#26834,.F.) ;
#37053=ORIENTED_EDGE('',*,*,#26838,.T.) ;
#37054=ORIENTED_EDGE('',*,*,#26838,.F.) ;
#37055=ORIENTED_EDGE('',*,*,#26836,.F.) ;
#37056=ORIENTED_EDGE('',*,*,#26833,.F.) ;
#37057=ORIENTED_EDGE('',*,*,#26667,.F.) ;
#37058=ORIENTED_EDGE('',*,*,#26839,.T.) ;
#37059=ORIENTED_EDGE('',*,*,#26840,.T.) ;
#37060=ORIENTED_EDGE('',*,*,#26664,.T.) ;
#37061=ORIENTED_EDGE('',*,*,#26841,.T.) ;
#37062=ORIENTED_EDGE('',*,*,#26842,.T.) ;
#37063=ORIENTED_EDGE('',*,*,#26843,.T.) ;
#37064=ORIENTED_EDGE('',*,*,#26839,.F.) ;
#37065=ORIENTED_EDGE('',*,*,#26844,.T.) ;
#37066=ORIENTED_EDGE('',*,*,#26662,.T.) ;
#37067=ORIENTED_EDGE('',*,*,#26845,.T.) ;
#37068=ORIENTED_EDGE('',*,*,#26842,.F.) ;
#37069=ORIENTED_EDGE('',*,*,#26846,.T.) ;
#37070=ORIENTED_EDGE('',*,*,#26846,.F.) ;
#37071=ORIENTED_EDGE('',*,*,#26844,.F.) ;
#37072=ORIENTED_EDGE('',*,*,#26841,.F.) ;
#37073=ORIENTED_EDGE('',*,*,#26663,.F.) ;
#37074=ORIENTED_EDGE('',*,*,#26847,.T.) ;
#37075=ORIENTED_EDGE('',*,*,#26848,.T.) ;
#37076=ORIENTED_EDGE('',*,*,#26676,.T.) ;
#37077=ORIENTED_EDGE('',*,*,#26849,.T.) ;
#37078=ORIENTED_EDGE('',*,*,#26850,.T.) ;
#37079=ORIENTED_EDGE('',*,*,#26851,.T.) ;
#37080=ORIENTED_EDGE('',*,*,#26847,.F.) ;
#37081=ORIENTED_EDGE('',*,*,#26852,.T.) ;
#37082=ORIENTED_EDGE('',*,*,#26674,.T.) ;
#37083=ORIENTED_EDGE('',*,*,#26853,.T.) ;
#37084=ORIENTED_EDGE('',*,*,#26850,.F.) ;
#37085=ORIENTED_EDGE('',*,*,#26854,.T.) ;
#37086=ORIENTED_EDGE('',*,*,#26854,.F.) ;
#37087=ORIENTED_EDGE('',*,*,#26852,.F.) ;
#37088=ORIENTED_EDGE('',*,*,#26849,.F.) ;
#37089=ORIENTED_EDGE('',*,*,#26675,.F.) ;
#37090=ORIENTED_EDGE('',*,*,#26855,.T.) ;
#37091=ORIENTED_EDGE('',*,*,#26856,.T.) ;
#37092=ORIENTED_EDGE('',*,*,#26672,.T.) ;
#37093=ORIENTED_EDGE('',*,*,#26857,.T.) ;
#37094=ORIENTED_EDGE('',*,*,#26858,.T.) ;
#37095=ORIENTED_EDGE('',*,*,#26859,.T.) ;
#37096=ORIENTED_EDGE('',*,*,#26855,.F.) ;
#37097=ORIENTED_EDGE('',*,*,#26860,.T.) ;
#37098=ORIENTED_EDGE('',*,*,#26670,.T.) ;
#37099=ORIENTED_EDGE('',*,*,#26861,.T.) ;
#37100=ORIENTED_EDGE('',*,*,#26858,.F.) ;
#37101=ORIENTED_EDGE('',*,*,#26862,.T.) ;
#37102=ORIENTED_EDGE('',*,*,#26862,.F.) ;
#37103=ORIENTED_EDGE('',*,*,#26860,.F.) ;
#37104=ORIENTED_EDGE('',*,*,#26857,.F.) ;
#37105=ORIENTED_EDGE('',*,*,#26671,.F.) ;
#37106=ORIENTED_EDGE('',*,*,#26863,.T.) ;
#37107=ORIENTED_EDGE('',*,*,#26864,.T.) ;
#37108=ORIENTED_EDGE('',*,*,#26653,.T.) ;
#37109=ORIENTED_EDGE('',*,*,#26865,.T.) ;
#37110=ORIENTED_EDGE('',*,*,#26866,.T.) ;
#37111=ORIENTED_EDGE('',*,*,#26867,.T.) ;
#37112=ORIENTED_EDGE('',*,*,#26863,.F.) ;
#37113=ORIENTED_EDGE('',*,*,#26868,.T.) ;
#37114=ORIENTED_EDGE('',*,*,#26659,.T.) ;
#37115=ORIENTED_EDGE('',*,*,#26869,.T.) ;
#37116=ORIENTED_EDGE('',*,*,#26866,.F.) ;
#37117=ORIENTED_EDGE('',*,*,#26870,.T.) ;
#37118=ORIENTED_EDGE('',*,*,#26870,.F.) ;
#37119=ORIENTED_EDGE('',*,*,#26868,.F.) ;
#37120=ORIENTED_EDGE('',*,*,#26865,.F.) ;
#37121=ORIENTED_EDGE('',*,*,#26660,.T.) ;
#37122=ORIENTED_EDGE('',*,*,#26871,.T.) ;
#37123=ORIENTED_EDGE('',*,*,#26872,.T.) ;
#37124=ORIENTED_EDGE('',*,*,#26657,.T.) ;
#37125=ORIENTED_EDGE('',*,*,#26873,.T.) ;
#37126=ORIENTED_EDGE('',*,*,#26874,.T.) ;
#37127=ORIENTED_EDGE('',*,*,#26875,.T.) ;
#37128=ORIENTED_EDGE('',*,*,#26871,.F.) ;
#37129=ORIENTED_EDGE('',*,*,#26876,.T.) ;
#37130=ORIENTED_EDGE('',*,*,#26655,.T.) ;
#37131=ORIENTED_EDGE('',*,*,#26877,.T.) ;
#37132=ORIENTED_EDGE('',*,*,#26874,.F.) ;
#37133=ORIENTED_EDGE('',*,*,#26878,.T.) ;
#37134=ORIENTED_EDGE('',*,*,#26878,.F.) ;
#37135=ORIENTED_EDGE('',*,*,#26876,.F.) ;
#37136=ORIENTED_EDGE('',*,*,#26873,.F.) ;
#37137=ORIENTED_EDGE('',*,*,#26656,.T.) ;
#37138=ORIENTED_EDGE('',*,*,#26869,.F.) ;
#37139=ORIENTED_EDGE('',*,*,#26658,.T.) ;
#37140=ORIENTED_EDGE('',*,*,#26872,.F.) ;
#37141=ORIENTED_EDGE('',*,*,#26879,.T.) ;
#37142=ORIENTED_EDGE('',*,*,#26867,.F.) ;
#37143=ORIENTED_EDGE('',*,*,#26879,.F.) ;
#37144=ORIENTED_EDGE('',*,*,#26875,.F.) ;
#37145=ORIENTED_EDGE('',*,*,#26880,.F.) ;
#37146=ORIENTED_EDGE('',*,*,#26864,.F.) ;
#37147=ORIENTED_EDGE('',*,*,#26880,.T.) ;
#37148=ORIENTED_EDGE('',*,*,#26877,.F.) ;
#37149=ORIENTED_EDGE('',*,*,#26654,.T.) ;
#37150=ORIENTED_EDGE('',*,*,#26853,.F.) ;
#37151=ORIENTED_EDGE('',*,*,#26673,.F.) ;
#37152=ORIENTED_EDGE('',*,*,#26856,.F.) ;
#37153=ORIENTED_EDGE('',*,*,#26881,.T.) ;
#37154=ORIENTED_EDGE('',*,*,#26851,.F.) ;
#37155=ORIENTED_EDGE('',*,*,#26881,.F.) ;
#37156=ORIENTED_EDGE('',*,*,#26859,.F.) ;
#37157=ORIENTED_EDGE('',*,*,#26882,.F.) ;
#37158=ORIENTED_EDGE('',*,*,#26848,.F.) ;
#37159=ORIENTED_EDGE('',*,*,#26882,.T.) ;
#37160=ORIENTED_EDGE('',*,*,#26861,.F.) ;
#37161=ORIENTED_EDGE('',*,*,#26669,.F.) ;
#37162=ORIENTED_EDGE('',*,*,#26832,.F.) ;
#37163=ORIENTED_EDGE('',*,*,#26883,.T.) ;
#37164=ORIENTED_EDGE('',*,*,#26845,.F.) ;
#37165=ORIENTED_EDGE('',*,*,#26661,.F.) ;
#37166=ORIENTED_EDGE('',*,*,#26835,.F.) ;
#37167=ORIENTED_EDGE('',*,*,#26884,.F.) ;
#37168=ORIENTED_EDGE('',*,*,#26843,.F.) ;
#37169=ORIENTED_EDGE('',*,*,#26883,.F.) ;
#37170=ORIENTED_EDGE('',*,*,#26837,.F.) ;
#37171=ORIENTED_EDGE('',*,*,#26665,.F.) ;
#37172=ORIENTED_EDGE('',*,*,#26840,.F.) ;
#37173=ORIENTED_EDGE('',*,*,#26884,.T.) ;
#37174=ORIENTED_EDGE('',*,*,#26816,.F.) ;
#37175=ORIENTED_EDGE('',*,*,#26885,.T.) ;
#37176=ORIENTED_EDGE('',*,*,#26829,.F.) ;
#37177=ORIENTED_EDGE('',*,*,#26681,.F.) ;
#37178=ORIENTED_EDGE('',*,*,#26819,.F.) ;
#37179=ORIENTED_EDGE('',*,*,#26886,.F.) ;
#37180=ORIENTED_EDGE('',*,*,#26827,.F.) ;
#37181=ORIENTED_EDGE('',*,*,#26885,.F.) ;
#37182=ORIENTED_EDGE('',*,*,#26821,.F.) ;
#37183=ORIENTED_EDGE('',*,*,#26677,.F.) ;
#37184=ORIENTED_EDGE('',*,*,#26824,.F.) ;
#37185=ORIENTED_EDGE('',*,*,#26886,.T.) ;
#37186=ORIENTED_EDGE('',*,*,#26887,.F.) ;
#37187=ORIENTED_EDGE('',*,*,#26888,.F.) ;
#37188=ORIENTED_EDGE('',*,*,#26889,.F.) ;
#37189=ORIENTED_EDGE('',*,*,#26890,.F.) ;
#37190=ORIENTED_EDGE('',*,*,#26890,.T.) ;
#37191=ORIENTED_EDGE('',*,*,#26891,.T.) ;
#37192=ORIENTED_EDGE('',*,*,#26719,.F.) ;
#37193=ORIENTED_EDGE('',*,*,#26892,.F.) ;
#37194=ORIENTED_EDGE('',*,*,#26889,.T.) ;
#37195=ORIENTED_EDGE('',*,*,#26893,.T.) ;
#37196=ORIENTED_EDGE('',*,*,#26720,.F.) ;
#37197=ORIENTED_EDGE('',*,*,#26891,.F.) ;
#37198=ORIENTED_EDGE('',*,*,#26611,.F.) ;
#37199=ORIENTED_EDGE('',*,*,#26648,.F.) ;
#37200=ORIENTED_EDGE('',*,*,#26894,.F.) ;
#37201=ORIENTED_EDGE('',*,*,#26691,.F.) ;
#37202=ORIENTED_EDGE('',*,*,#26619,.F.) ;
#37203=ORIENTED_EDGE('',*,*,#26804,.F.) ;
#37204=ORIENTED_EDGE('',*,*,#26894,.T.) ;
#37205=ORIENTED_EDGE('',*,*,#26647,.F.) ;
#37206=ORIENTED_EDGE('',*,*,#26895,.T.) ;
#37207=ORIENTED_EDGE('',*,*,#26692,.F.) ;
#37208=ORIENTED_EDGE('',*,*,#26792,.F.) ;
#37209=ORIENTED_EDGE('',*,*,#26795,.T.) ;
#37210=ORIENTED_EDGE('',*,*,#26717,.F.) ;
#37211=ORIENTED_EDGE('',*,*,#26896,.F.) ;
#37212=ORIENTED_EDGE('',*,*,#26790,.F.) ;
#37213=ORIENTED_EDGE('',*,*,#26896,.T.) ;
#37214=ORIENTED_EDGE('',*,*,#26716,.F.) ;
#37215=ORIENTED_EDGE('',*,*,#26796,.F.) ;
#37216=ORIENTED_EDGE('',*,*,#26888,.T.) ;
#37217=ORIENTED_EDGE('',*,*,#26897,.T.) ;
#37218=ORIENTED_EDGE('',*,*,#26721,.F.) ;
#37219=ORIENTED_EDGE('',*,*,#26893,.F.) ;
#37220=ORIENTED_EDGE('',*,*,#26887,.T.) ;
#37221=ORIENTED_EDGE('',*,*,#26892,.T.) ;
#37222=ORIENTED_EDGE('',*,*,#26718,.F.) ;
#37223=ORIENTED_EDGE('',*,*,#26897,.F.) ;
#37224=ORIENTED_EDGE('',*,*,#26722,.F.) ;
#37225=ORIENTED_EDGE('',*,*,#26698,.F.) ;
#37226=ORIENTED_EDGE('',*,*,#26898,.F.) ;
#37227=ORIENTED_EDGE('',*,*,#26641,.T.) ;
#37228=ORIENTED_EDGE('',*,*,#26725,.F.) ;
#37229=ORIENTED_EDGE('',*,*,#26728,.T.) ;
#37230=ORIENTED_EDGE('',*,*,#26642,.T.) ;
#37231=ORIENTED_EDGE('',*,*,#26898,.T.) ;
#37232=ORIENTED_EDGE('',*,*,#26697,.F.) ;
#37233=ORIENTED_EDGE('',*,*,#26899,.F.) ;
#37234=ORIENTED_EDGE('',*,*,#26643,.T.) ;
#37235=ORIENTED_EDGE('',*,*,#26899,.T.) ;
#37236=ORIENTED_EDGE('',*,*,#26696,.F.) ;
#37237=ORIENTED_EDGE('',*,*,#26900,.F.) ;
#37238=ORIENTED_EDGE('',*,*,#26644,.T.) ;
#37239=ORIENTED_EDGE('',*,*,#26900,.T.) ;
#37240=ORIENTED_EDGE('',*,*,#26695,.F.) ;
#37241=ORIENTED_EDGE('',*,*,#26901,.F.) ;
#37242=ORIENTED_EDGE('',*,*,#26645,.T.) ;
#37243=ORIENTED_EDGE('',*,*,#26901,.T.) ;
#37244=ORIENTED_EDGE('',*,*,#26694,.F.) ;
#37245=ORIENTED_EDGE('',*,*,#26902,.F.) ;
#37246=ORIENTED_EDGE('',*,*,#26646,.T.) ;
#37247=ORIENTED_EDGE('',*,*,#26902,.T.) ;
#37248=ORIENTED_EDGE('',*,*,#26693,.F.) ;
#37249=ORIENTED_EDGE('',*,*,#26895,.F.) ;
#45668=TOROIDAL_SURFACE('',#51776,0.4,0.1) ;
#45669=TOROIDAL_SURFACE('',#51780,0.4,0.1) ;
#45670=TOROIDAL_SURFACE('',#51790,0.4,0.1) ;
#45671=TOROIDAL_SURFACE('',#51794,0.4,0.1) ;
#45672=TOROIDAL_SURFACE('',#51800,0.4,0.1) ;
#45673=TOROIDAL_SURFACE('',#51804,0.4,0.1) ;
#45674=TOROIDAL_SURFACE('',#51838,1.55266329058736,0.1) ;
#45675=TOROIDAL_SURFACE('',#51843,1.55266329058736,0.1) ;
#45676=TOROIDAL_SURFACE('',#51847,3.1,0.1) ;
#45677=TOROIDAL_SURFACE('',#51853,3.1,0.1) ;
#45678=TOROIDAL_SURFACE('',#51867,0.899999999999993,0.3) ;
#45679=TOROIDAL_SURFACE('',#51873,0.899999999999993,0.3) ;
#45680=TOROIDAL_SURFACE('',#51877,0.899999999999993,0.3) ;
#45681=TOROIDAL_SURFACE('',#51883,0.899999999999993,0.3) ;
#45682=TOROIDAL_SURFACE('',#51887,0.899999999999993,0.3) ;
#45683=TOROIDAL_SURFACE('',#51893,0.899999999999993,0.3) ;
#45684=TOROIDAL_SURFACE('',#51897,0.899999999999993,0.3) ;
#45685=TOROIDAL_SURFACE('',#51903,0.899999999999993,0.3) ;
#45686=TOROIDAL_SURFACE('',#51907,0.899999999999993,0.3) ;
#45687=TOROIDAL_SURFACE('',#51913,0.899999999999993,0.3) ;
#45688=TOROIDAL_SURFACE('',#51917,0.899999999999993,0.3) ;
#45689=TOROIDAL_SURFACE('',#51923,0.899999999999993,0.3) ;
#45690=TOROIDAL_SURFACE('',#51927,0.899999999999993,0.3) ;
#45691=TOROIDAL_SURFACE('',#51933,0.899999999999993,0.3) ;
#45692=TOROIDAL_SURFACE('',#51937,0.899999999999993,0.3) ;
#45693=TOROIDAL_SURFACE('',#51943,0.899999999999993,0.3) ;
#47194=ADVANCED_FACE('',(#11976),#9939,.T.) ;
#47195=ADVANCED_FACE('',(#11977),#9940,.T.) ;
#47196=ADVANCED_FACE('',(#11978),#9941,.T.) ;
#47197=ADVANCED_FACE('',(#11979),#2193,.T.) ;
#47198=ADVANCED_FACE('',(#11980),#2194,.T.) ;
#47199=ADVANCED_FACE('',(#11981,#722,#723,#724,#725,#726),#2435,.F.) ;
#47200=ADVANCED_FACE('',(#11982),#9942,.T.) ;
#47201=ADVANCED_FACE('',(#11983),#2436,.T.) ;
#47202=ADVANCED_FACE('',(#11984),#9943,.T.) ;
#47203=ADVANCED_FACE('',(#11985,#727,#728),#2437,.T.) ;
#47204=ADVANCED_FACE('',(#11986),#9944,.T.) ;
#47205=ADVANCED_FACE('',(#11987),#9945,.T.) ;
#47206=ADVANCED_FACE('',(#11988),#2438,.T.) ;
#47207=ADVANCED_FACE('',(#11989),#45668,.T.) ;
#47208=ADVANCED_FACE('',(#11990),#45669,.T.) ;
#47209=ADVANCED_FACE('',(#11991),#9946,.T.) ;
#47210=ADVANCED_FACE('',(#11992),#2439,.T.) ;
#47211=ADVANCED_FACE('',(#11993),#9947,.T.) ;
#47212=ADVANCED_FACE('',(#11994),#9948,.T.) ;
#47213=ADVANCED_FACE('',(#11995),#45670,.T.) ;
#47214=ADVANCED_FACE('',(#11996),#45671,.T.) ;
#47215=ADVANCED_FACE('',(#11997),#9949,.T.) ;
#47216=ADVANCED_FACE('',(#11998),#9950,.T.) ;
#47217=ADVANCED_FACE('',(#11999),#2440,.T.) ;
#47218=ADVANCED_FACE('',(#12000),#45672,.T.) ;
#47219=ADVANCED_FACE('',(#12001),#45673,.T.) ;
#47220=ADVANCED_FACE('',(#12002),#9951,.T.) ;
#47221=ADVANCED_FACE('',(#12003),#9952,.T.) ;
#47222=ADVANCED_FACE('',(#12004),#2441,.T.) ;
#47223=ADVANCED_FACE('',(#12005),#9953,.T.) ;
#47224=ADVANCED_FACE('',(#12006),#1989,.T.) ;
#47225=ADVANCED_FACE('',(#12007),#9954,.F.) ;
#47226=ADVANCED_FACE('',(#12008),#1990,.T.) ;
#47227=ADVANCED_FACE('',(#12009),#2442,.T.) ;
#47228=ADVANCED_FACE('',(#12010),#9955,.T.) ;
#47229=ADVANCED_FACE('',(#12011),#9956,.T.) ;
#47230=ADVANCED_FACE('',(#12012),#95,.F.) ;
#47231=ADVANCED_FACE('',(#12013),#96,.F.) ;
#47232=ADVANCED_FACE('',(#12014),#9957,.T.) ;
#47233=ADVANCED_FACE('',(#12015),#9958,.T.) ;
#47234=ADVANCED_FACE('',(#12016),#2443,.T.) ;
#47235=ADVANCED_FACE('',(#12017),#9959,.T.) ;
#47236=ADVANCED_FACE('',(#12018),#45674,.T.) ;
#47237=ADVANCED_FACE('',(#12019),#9960,.T.) ;
#47238=ADVANCED_FACE('',(#12020),#45675,.T.) ;
#47239=ADVANCED_FACE('',(#12021),#9961,.F.) ;
#47240=ADVANCED_FACE('',(#12022),#2444,.T.) ;
#47241=ADVANCED_FACE('',(#12023),#45676,.T.) ;
#47242=ADVANCED_FACE('',(#12024),#2445,.T.) ;
#47243=ADVANCED_FACE('',(#12025),#9962,.F.) ;
#47244=ADVANCED_FACE('',(#12026),#2446,.T.) ;
#47245=ADVANCED_FACE('',(#12027),#45677,.T.) ;
#47246=ADVANCED_FACE('',(#12028),#2447,.T.) ;
#47247=ADVANCED_FACE('',(#12029),#9963,.T.) ;
#47248=ADVANCED_FACE('',(#12030),#9964,.T.) ;
#47249=ADVANCED_FACE('',(#12031),#9965,.T.) ;
#47250=ADVANCED_FACE('',(#12032),#9966,.T.) ;
#47251=ADVANCED_FACE('',(#12033),#2448,.T.) ;
#47252=ADVANCED_FACE('',(#12034),#2449,.T.) ;
#47253=ADVANCED_FACE('',(#12035),#2450,.T.) ;
#47254=ADVANCED_FACE('',(#12036),#9967,.T.) ;
#47255=ADVANCED_FACE('',(#12037),#9968,.T.) ;
#47256=ADVANCED_FACE('',(#12038),#45678,.T.) ;
#47257=ADVANCED_FACE('',(#12039),#9969,.T.) ;
#47258=ADVANCED_FACE('',(#12040),#45679,.T.) ;
#47259=ADVANCED_FACE('',(#12041),#2451,.T.) ;
#47260=ADVANCED_FACE('',(#12042),#45680,.T.) ;
#47261=ADVANCED_FACE('',(#12043),#9970,.T.) ;
#47262=ADVANCED_FACE('',(#12044),#45681,.T.) ;
#47263=ADVANCED_FACE('',(#12045),#2452,.T.) ;
#47264=ADVANCED_FACE('',(#12046),#45682,.T.) ;
#47265=ADVANCED_FACE('',(#12047),#9971,.T.) ;
#47266=ADVANCED_FACE('',(#12048),#45683,.T.) ;
#47267=ADVANCED_FACE('',(#12049),#2453,.T.) ;
#47268=ADVANCED_FACE('',(#12050),#45684,.T.) ;
#47269=ADVANCED_FACE('',(#12051),#9972,.T.) ;
#47270=ADVANCED_FACE('',(#12052),#45685,.T.) ;
#47271=ADVANCED_FACE('',(#12053),#2454,.T.) ;
#47272=ADVANCED_FACE('',(#12054),#45686,.T.) ;
#47273=ADVANCED_FACE('',(#12055),#9973,.T.) ;
#47274=ADVANCED_FACE('',(#12056),#45687,.T.) ;
#47275=ADVANCED_FACE('',(#12057),#2455,.T.) ;
#47276=ADVANCED_FACE('',(#12058),#45688,.T.) ;
#47277=ADVANCED_FACE('',(#12059),#9974,.T.) ;
#47278=ADVANCED_FACE('',(#12060),#45689,.T.) ;
#47279=ADVANCED_FACE('',(#12061),#2456,.T.) ;
#47280=ADVANCED_FACE('',(#12062),#45690,.T.) ;
#47281=ADVANCED_FACE('',(#12063),#9975,.T.) ;
#47282=ADVANCED_FACE('',(#12064),#45691,.T.) ;
#47283=ADVANCED_FACE('',(#12065),#2457,.T.) ;
#47284=ADVANCED_FACE('',(#12066),#45692,.T.) ;
#47285=ADVANCED_FACE('',(#12067),#9976,.T.) ;
#47286=ADVANCED_FACE('',(#12068),#45693,.T.) ;
#47287=ADVANCED_FACE('',(#12069),#2458,.T.) ;
#47288=ADVANCED_FACE('',(#12070),#9977,.T.) ;
#47289=ADVANCED_FACE('',(#12071),#2459,.T.) ;
#47290=ADVANCED_FACE('',(#12072),#9978,.T.) ;
#47291=ADVANCED_FACE('',(#12073),#9979,.T.) ;
#47292=ADVANCED_FACE('',(#12074),#2460,.T.) ;
#47293=ADVANCED_FACE('',(#12075),#9980,.T.) ;
#47294=ADVANCED_FACE('',(#12076),#9981,.T.) ;
#47295=ADVANCED_FACE('',(#12077),#2461,.T.) ;
#47296=ADVANCED_FACE('',(#12078),#9982,.T.) ;
#47297=ADVANCED_FACE('',(#12079),#9983,.T.) ;
#47298=ADVANCED_FACE('',(#12080),#2462,.T.) ;
#47299=ADVANCED_FACE('',(#12081),#9984,.T.) ;
#47300=ADVANCED_FACE('',(#12082),#2463,.T.) ;
#47301=ADVANCED_FACE('',(#12083),#2464,.T.) ;
#47302=ADVANCED_FACE('',(#12084),#2465,.T.) ;
#47303=ADVANCED_FACE('',(#12085),#9985,.F.) ;
#47304=ADVANCED_FACE('',(#12086),#2466,.T.) ;
#47305=ADVANCED_FACE('',(#12087),#2467,.T.) ;
#47306=ADVANCED_FACE('',(#12088),#9986,.F.) ;
#47307=ADVANCED_FACE('',(#12089),#2468,.T.) ;
#47308=ADVANCED_FACE('',(#12090),#2469,.T.) ;
#47309=ADVANCED_FACE('',(#12091),#2470,.T.) ;
#47310=ADVANCED_FACE('',(#12092),#2471,.T.) ;
#47311=ADVANCED_FACE('',(#12093),#2472,.T.) ;
#47312=ADVANCED_FACE('',(#12094),#2473,.T.) ;
#47313=ADVANCED_FACE('',(#12095),#2474,.T.) ;
#47314=ADVANCED_FACE('',(#12096),#2475,.T.) ;
#49061=CLOSED_SHELL('',(#47194,#47195,#47196,#47197,#47198,#47199,#47200,
#47201,#47202,#47203,#47204,#47205,#47206,#47207,#47208,#47209,#47210,#47211,
#47212,#47213,#47214,#47215,#47216,#47217,#47218,#47219,#47220,#47221,#47222,
#47223,#47224,#47225,#47226,#47227,#47228,#47229,#47230,#47231,#47232,#47233,
#47234,#47235,#47236,#47237,#47238,#47239,#47240,#47241,#47242,#47243,#47244,
#47245,#47246,#47247,#47248,#47249,#47250,#47251,#47252,#47253,#47254,#47255,
#47256,#47257,#47258,#47259,#47260,#47261,#47262,#47263,#47264,#47265,#47266,
#47267,#47268,#47269,#47270,#47271,#47272,#47273,#47274,#47275,#47276,#47277,
#47278,#47279,#47280,#47281,#47282,#47283,#47284,#47285,#47286,#47287,#47288,
#47289,#47290,#47291,#47292,#47293,#47294,#47295,#47296,#47297,#47298,#47299,
#47300,#47301,#47302,#47303,#47304,#47305,#47306,#47307,#47308,#47309,#47310,
#47311,#47312,#47313,#47314)) ;
#51734=AXIS2_PLACEMENT_3D('',#86611,#61018,#61019) ;
#51735=AXIS2_PLACEMENT_3D('',#86612,#61020,#61021) ;
#51736=AXIS2_PLACEMENT_3D('',#86628,#61023,#61024) ;
#51737=AXIS2_PLACEMENT_3D('',#86630,#61026,#61027) ;
#51738=AXIS2_PLACEMENT_3D('',#86632,#61028,#61029) ;
#51739=AXIS2_PLACEMENT_3D('',#86636,#61031,#61032) ;
#51740=AXIS2_PLACEMENT_3D('',#86638,#61034,#61035) ;
#51741=AXIS2_PLACEMENT_3D('',#86653,#61037,#61038) ;
#51742=AXIS2_PLACEMENT_3D('',#86655,#61040,#61041) ;
#51743=AXIS2_PLACEMENT_3D('',#86656,#61042,#61043) ;
#51744=AXIS2_PLACEMENT_3D('',#86657,#61044,#61045) ;
#51745=AXIS2_PLACEMENT_3D('',#86658,#61046,#61047) ;
#51746=AXIS2_PLACEMENT_3D('',#86659,#61048,#61049) ;
#51747=AXIS2_PLACEMENT_3D('',#86663,#61051,#61052) ;
#51748=AXIS2_PLACEMENT_3D('',#86675,#61058,#61059) ;
#51749=AXIS2_PLACEMENT_3D('',#86679,#61061,#61062) ;
#51750=AXIS2_PLACEMENT_3D('',#86683,#61064,#61065) ;
#51751=AXIS2_PLACEMENT_3D('',#86687,#61067,#61068) ;
#51752=AXIS2_PLACEMENT_3D('',#86706,#61078,#61079) ;
#51753=AXIS2_PLACEMENT_3D('',#86711,#61081,#61082) ;
#51754=AXIS2_PLACEMENT_3D('',#86714,#61084,#61085) ;
#51755=AXIS2_PLACEMENT_3D('',#86923,#61102,#61103) ;
#51756=AXIS2_PLACEMENT_3D('',#86926,#61105,#61106) ;
#51757=AXIS2_PLACEMENT_3D('',#86927,#61107,#61108) ;
#51758=AXIS2_PLACEMENT_3D('',#86931,#61111,#61112) ;
#51759=AXIS2_PLACEMENT_3D('',#86934,#61114,#61115) ;
#51760=AXIS2_PLACEMENT_3D('',#86935,#61116,#61117) ;
#51761=AXIS2_PLACEMENT_3D('',#86937,#61118,#61119) ;
#51762=AXIS2_PLACEMENT_3D('',#86957,#61129,#61130) ;
#51763=AXIS2_PLACEMENT_3D('',#86961,#61132,#61133) ;
#51764=AXIS2_PLACEMENT_3D('',#86965,#61135,#61136) ;
#51765=AXIS2_PLACEMENT_3D('',#86969,#61138,#61139) ;
#51766=AXIS2_PLACEMENT_3D('',#86980,#61145,#61146) ;
#51767=AXIS2_PLACEMENT_3D('',#86983,#61147,#61148) ;
#51768=AXIS2_PLACEMENT_3D('',#86987,#61150,#61151) ;
#51769=AXIS2_PLACEMENT_3D('',#86997,#61157,#61158) ;
#51770=AXIS2_PLACEMENT_3D('',#86999,#61159,#61160) ;
#51771=AXIS2_PLACEMENT_3D('',#87002,#61162,#61163) ;
#51772=AXIS2_PLACEMENT_3D('',#87003,#61164,#61165) ;
#51773=AXIS2_PLACEMENT_3D('',#87005,#61166,#61167) ;
#51774=AXIS2_PLACEMENT_3D('',#87007,#61168,#61169) ;
#51775=AXIS2_PLACEMENT_3D('',#87009,#61171,#61172) ;
#51776=AXIS2_PLACEMENT_3D('',#87012,#61175,#61176) ;
#51777=AXIS2_PLACEMENT_3D('',#87014,#61177,#61178) ;
#51778=AXIS2_PLACEMENT_3D('',#87016,#61179,#61180) ;
#51779=AXIS2_PLACEMENT_3D('',#87017,#61181,#61182) ;
#51780=AXIS2_PLACEMENT_3D('',#87018,#61183,#61184) ;
#51781=AXIS2_PLACEMENT_3D('',#87020,#61185,#61186) ;
#51782=AXIS2_PLACEMENT_3D('',#87022,#61187,#61188) ;
#51783=AXIS2_PLACEMENT_3D('',#87023,#61189,#61190) ;
#51784=AXIS2_PLACEMENT_3D('',#87024,#61191,#61192) ;
#51785=AXIS2_PLACEMENT_3D('',#87027,#61195,#61196) ;
#51786=AXIS2_PLACEMENT_3D('',#87033,#61200,#61201) ;
#51787=AXIS2_PLACEMENT_3D('',#87034,#61202,#61203) ;
#51788=AXIS2_PLACEMENT_3D('',#87035,#61204,#61205) ;
#51789=AXIS2_PLACEMENT_3D('',#87038,#61207,#61208) ;
#51790=AXIS2_PLACEMENT_3D('',#87039,#61209,#61210) ;
#51791=AXIS2_PLACEMENT_3D('',#87041,#61211,#61212) ;
#51792=AXIS2_PLACEMENT_3D('',#87043,#61213,#61214) ;
#51793=AXIS2_PLACEMENT_3D('',#87044,#61215,#61216) ;
#51794=AXIS2_PLACEMENT_3D('',#87045,#61217,#61218) ;
#51795=AXIS2_PLACEMENT_3D('',#87047,#61219,#61220) ;
#51796=AXIS2_PLACEMENT_3D('',#87048,#61221,#61222) ;
#51797=AXIS2_PLACEMENT_3D('',#87049,#61223,#61224) ;
#51798=AXIS2_PLACEMENT_3D('',#87052,#61227,#61228) ;
#51799=AXIS2_PLACEMENT_3D('',#87054,#61230,#61231) ;
#51800=AXIS2_PLACEMENT_3D('',#87055,#61232,#61233) ;
#51801=AXIS2_PLACEMENT_3D('',#87057,#61234,#61235) ;
#51802=AXIS2_PLACEMENT_3D('',#87058,#61236,#61237) ;
#51803=AXIS2_PLACEMENT_3D('',#87059,#61238,#61239) ;
#51804=AXIS2_PLACEMENT_3D('',#87060,#61240,#61241) ;
#51805=AXIS2_PLACEMENT_3D('',#87062,#61242,#61243) ;
#51806=AXIS2_PLACEMENT_3D('',#87063,#61244,#61245) ;
#51807=AXIS2_PLACEMENT_3D('',#87064,#61246,#61247) ;
#51808=AXIS2_PLACEMENT_3D('',#87066,#61249,#61250) ;
#51809=AXIS2_PLACEMENT_3D('',#87069,#61252,#61253) ;
#51810=AXIS2_PLACEMENT_3D('',#87070,#61254,#61255) ;
#51811=AXIS2_PLACEMENT_3D('',#87074,#61258,#61259) ;
#51812=AXIS2_PLACEMENT_3D('',#87075,#61260,#61261) ;
#51813=AXIS2_PLACEMENT_3D('',#87103,#61262,#61263) ;
#51814=AXIS2_PLACEMENT_3D('',#87105,#61264,#61265) ;
#51815=AXIS2_PLACEMENT_3D('',#87106,#61266,#61267) ;
#51816=AXIS2_PLACEMENT_3D('',#87108,#61268,#61269) ;
#51817=AXIS2_PLACEMENT_3D('',#87109,#61270,#61271) ;
#51818=AXIS2_PLACEMENT_3D('',#87110,#61272,#61273) ;
#51819=AXIS2_PLACEMENT_3D('',#87114,#61275,#61276) ;
#51820=AXIS2_PLACEMENT_3D('',#87142,#61278,#61279) ;
#51821=AXIS2_PLACEMENT_3D('',#87143,#61280,#61281) ;
#51822=AXIS2_PLACEMENT_3D('',#87145,#61282,#61283) ;
#51823=AXIS2_PLACEMENT_3D('',#87146,#61284,#61285) ;
#51824=AXIS2_PLACEMENT_3D('',#87147,#61286,#61287) ;
#51825=AXIS2_PLACEMENT_3D('',#87153,#61291,#61292) ;
#51826=AXIS2_PLACEMENT_3D('',#87154,#61293,#61294) ;
#51827=AXIS2_PLACEMENT_3D('',#87155,#61295,#61296) ;
#51828=AXIS2_PLACEMENT_3D('',#87158,#61298,#61299) ;
#51829=AXIS2_PLACEMENT_3D('',#87169,#61300,#61301) ;
#51830=AXIS2_PLACEMENT_3D('',#87170,#61302,#61303) ;
#51831=AXIS2_PLACEMENT_3D('',#87180,#61304,#61305) ;
#51832=AXIS2_PLACEMENT_3D('',#87181,#61306,#61307) ;
#51833=AXIS2_PLACEMENT_3D('',#87183,#61309,#61310) ;
#51834=AXIS2_PLACEMENT_3D('',#87185,#61312,#61313) ;
#51835=AXIS2_PLACEMENT_3D('',#87186,#61314,#61315) ;
#51836=AXIS2_PLACEMENT_3D('',#87188,#61316,#61317) ;
#51837=AXIS2_PLACEMENT_3D('',#87190,#61318,#61319) ;
#51838=AXIS2_PLACEMENT_3D('',#87192,#61321,#61322) ;
#51839=AXIS2_PLACEMENT_3D('',#87194,#61323,#61324) ;
#51840=AXIS2_PLACEMENT_3D('',#87195,#61325,#61326) ;
#51841=AXIS2_PLACEMENT_3D('',#87196,#61327,#61328) ;
#51842=AXIS2_PLACEMENT_3D('',#87198,#61329,#61330) ;
#51843=AXIS2_PLACEMENT_3D('',#87200,#61332,#61333) ;
#51844=AXIS2_PLACEMENT_3D('',#87201,#61334,#61335) ;
#51845=AXIS2_PLACEMENT_3D('',#87202,#61336,#61337) ;
#51846=AXIS2_PLACEMENT_3D('',#87205,#61340,#61341) ;
#51847=AXIS2_PLACEMENT_3D('',#87207,#61343,#61344) ;
#51848=AXIS2_PLACEMENT_3D('',#87216,#61345,#61346) ;
#51849=AXIS2_PLACEMENT_3D('',#87221,#61347,#61348) ;
#51850=AXIS2_PLACEMENT_3D('',#87230,#61351,#61352) ;
#51851=AXIS2_PLACEMENT_3D('',#87231,#61353,#61354) ;
#51852=AXIS2_PLACEMENT_3D('',#87232,#61355,#61356) ;
#51853=AXIS2_PLACEMENT_3D('',#87234,#61358,#61359) ;
#51854=AXIS2_PLACEMENT_3D('',#87241,#61360,#61361) ;
#51855=AXIS2_PLACEMENT_3D('',#87243,#61363,#61364) ;
#51856=AXIS2_PLACEMENT_3D('',#87246,#61366,#61367) ;
#51857=AXIS2_PLACEMENT_3D('',#87247,#61368,#61369) ;
#51858=AXIS2_PLACEMENT_3D('',#87248,#61370,#61371) ;
#51859=AXIS2_PLACEMENT_3D('',#87249,#61372,#61373) ;
#51860=AXIS2_PLACEMENT_3D('',#87250,#61374,#61375) ;
#51861=AXIS2_PLACEMENT_3D('',#87252,#61377,#61378) ;
#51862=AXIS2_PLACEMENT_3D('',#87255,#61380,#61381) ;
#51863=AXIS2_PLACEMENT_3D('',#87256,#61382,#61383) ;
#51864=AXIS2_PLACEMENT_3D('',#87258,#61385,#61386) ;
#51865=AXIS2_PLACEMENT_3D('',#87260,#61388,#61389) ;
#51866=AXIS2_PLACEMENT_3D('',#87261,#61390,#61391) ;
#51867=AXIS2_PLACEMENT_3D('',#87262,#61392,#61393) ;
#51868=AXIS2_PLACEMENT_3D('',#87265,#61394,#61395) ;
#51869=AXIS2_PLACEMENT_3D('',#87266,#61396,#61397) ;
#51870=AXIS2_PLACEMENT_3D('',#87267,#61398,#61399) ;
#51871=AXIS2_PLACEMENT_3D('',#87268,#61400,#61401) ;
#51872=AXIS2_PLACEMENT_3D('',#87271,#61402,#61403) ;
#51873=AXIS2_PLACEMENT_3D('',#87274,#61406,#61407) ;
#51874=AXIS2_PLACEMENT_3D('',#87275,#61408,#61409) ;
#51875=AXIS2_PLACEMENT_3D('',#87276,#61410,#61411) ;
#51876=AXIS2_PLACEMENT_3D('',#87277,#61412,#61413) ;
#51877=AXIS2_PLACEMENT_3D('',#87278,#61414,#61415) ;
#51878=AXIS2_PLACEMENT_3D('',#87281,#61416,#61417) ;
#51879=AXIS2_PLACEMENT_3D('',#87282,#61418,#61419) ;
#51880=AXIS2_PLACEMENT_3D('',#87283,#61420,#61421) ;
#51881=AXIS2_PLACEMENT_3D('',#87284,#61422,#61423) ;
#51882=AXIS2_PLACEMENT_3D('',#87287,#61424,#61425) ;
#51883=AXIS2_PLACEMENT_3D('',#87290,#61428,#61429) ;
#51884=AXIS2_PLACEMENT_3D('',#87291,#61430,#61431) ;
#51885=AXIS2_PLACEMENT_3D('',#87292,#61432,#61433) ;
#51886=AXIS2_PLACEMENT_3D('',#87293,#61434,#61435) ;
#51887=AXIS2_PLACEMENT_3D('',#87294,#61436,#61437) ;
#51888=AXIS2_PLACEMENT_3D('',#87297,#61438,#61439) ;
#51889=AXIS2_PLACEMENT_3D('',#87298,#61440,#61441) ;
#51890=AXIS2_PLACEMENT_3D('',#87299,#61442,#61443) ;
#51891=AXIS2_PLACEMENT_3D('',#87300,#61444,#61445) ;
#51892=AXIS2_PLACEMENT_3D('',#87303,#61446,#61447) ;
#51893=AXIS2_PLACEMENT_3D('',#87306,#61450,#61451) ;
#51894=AXIS2_PLACEMENT_3D('',#87307,#61452,#61453) ;
#51895=AXIS2_PLACEMENT_3D('',#87308,#61454,#61455) ;
#51896=AXIS2_PLACEMENT_3D('',#87309,#61456,#61457) ;
#51897=AXIS2_PLACEMENT_3D('',#87310,#61458,#61459) ;
#51898=AXIS2_PLACEMENT_3D('',#87313,#61460,#61461) ;
#51899=AXIS2_PLACEMENT_3D('',#87314,#61462,#61463) ;
#51900=AXIS2_PLACEMENT_3D('',#87315,#61464,#61465) ;
#51901=AXIS2_PLACEMENT_3D('',#87316,#61466,#61467) ;
#51902=AXIS2_PLACEMENT_3D('',#87319,#61468,#61469) ;
#51903=AXIS2_PLACEMENT_3D('',#87322,#61472,#61473) ;
#51904=AXIS2_PLACEMENT_3D('',#87323,#61474,#61475) ;
#51905=AXIS2_PLACEMENT_3D('',#87324,#61476,#61477) ;
#51906=AXIS2_PLACEMENT_3D('',#87325,#61478,#61479) ;
#51907=AXIS2_PLACEMENT_3D('',#87326,#61480,#61481) ;
#51908=AXIS2_PLACEMENT_3D('',#87329,#61482,#61483) ;
#51909=AXIS2_PLACEMENT_3D('',#87330,#61484,#61485) ;
#51910=AXIS2_PLACEMENT_3D('',#87331,#61486,#61487) ;
#51911=AXIS2_PLACEMENT_3D('',#87332,#61488,#61489) ;
#51912=AXIS2_PLACEMENT_3D('',#87335,#61490,#61491) ;
#51913=AXIS2_PLACEMENT_3D('',#87338,#61494,#61495) ;
#51914=AXIS2_PLACEMENT_3D('',#87339,#61496,#61497) ;
#51915=AXIS2_PLACEMENT_3D('',#87340,#61498,#61499) ;
#51916=AXIS2_PLACEMENT_3D('',#87341,#61500,#61501) ;
#51917=AXIS2_PLACEMENT_3D('',#87342,#61502,#61503) ;
#51918=AXIS2_PLACEMENT_3D('',#87345,#61504,#61505) ;
#51919=AXIS2_PLACEMENT_3D('',#87346,#61506,#61507) ;
#51920=AXIS2_PLACEMENT_3D('',#87347,#61508,#61509) ;
#51921=AXIS2_PLACEMENT_3D('',#87348,#61510,#61511) ;
#51922=AXIS2_PLACEMENT_3D('',#87351,#61512,#61513) ;
#51923=AXIS2_PLACEMENT_3D('',#87354,#61516,#61517) ;
#51924=AXIS2_PLACEMENT_3D('',#87355,#61518,#61519) ;
#51925=AXIS2_PLACEMENT_3D('',#87356,#61520,#61521) ;
#51926=AXIS2_PLACEMENT_3D('',#87357,#61522,#61523) ;
#51927=AXIS2_PLACEMENT_3D('',#87358,#61524,#61525) ;
#51928=AXIS2_PLACEMENT_3D('',#87361,#61526,#61527) ;
#51929=AXIS2_PLACEMENT_3D('',#87362,#61528,#61529) ;
#51930=AXIS2_PLACEMENT_3D('',#87363,#61530,#61531) ;
#51931=AXIS2_PLACEMENT_3D('',#87364,#61532,#61533) ;
#51932=AXIS2_PLACEMENT_3D('',#87367,#61534,#61535) ;
#51933=AXIS2_PLACEMENT_3D('',#87370,#61538,#61539) ;
#51934=AXIS2_PLACEMENT_3D('',#87371,#61540,#61541) ;
#51935=AXIS2_PLACEMENT_3D('',#87372,#61542,#61543) ;
#51936=AXIS2_PLACEMENT_3D('',#87373,#61544,#61545) ;
#51937=AXIS2_PLACEMENT_3D('',#87374,#61546,#61547) ;
#51938=AXIS2_PLACEMENT_3D('',#87377,#61548,#61549) ;
#51939=AXIS2_PLACEMENT_3D('',#87378,#61550,#61551) ;
#51940=AXIS2_PLACEMENT_3D('',#87379,#61552,#61553) ;
#51941=AXIS2_PLACEMENT_3D('',#87380,#61554,#61555) ;
#51942=AXIS2_PLACEMENT_3D('',#87383,#61556,#61557) ;
#51943=AXIS2_PLACEMENT_3D('',#87386,#61560,#61561) ;
#51944=AXIS2_PLACEMENT_3D('',#87387,#61562,#61563) ;
#51945=AXIS2_PLACEMENT_3D('',#87388,#61564,#61565) ;
#51946=AXIS2_PLACEMENT_3D('',#87389,#61566,#61567) ;
#51947=AXIS2_PLACEMENT_3D('',#87390,#61568,#61569) ;
#51948=AXIS2_PLACEMENT_3D('',#87392,#61571,#61572) ;
#51949=AXIS2_PLACEMENT_3D('',#87394,#61574,#61575) ;
#51950=AXIS2_PLACEMENT_3D('',#87395,#61576,#61577) ;
#51951=AXIS2_PLACEMENT_3D('',#87397,#61579,#61580) ;
#51952=AXIS2_PLACEMENT_3D('',#87399,#61582,#61583) ;
#51953=AXIS2_PLACEMENT_3D('',#87400,#61584,#61585) ;
#51954=AXIS2_PLACEMENT_3D('',#87402,#61587,#61588) ;
#51955=AXIS2_PLACEMENT_3D('',#87404,#61590,#61591) ;
#51956=AXIS2_PLACEMENT_3D('',#87405,#61592,#61593) ;
#51957=AXIS2_PLACEMENT_3D('',#87407,#61595,#61596) ;
#51958=AXIS2_PLACEMENT_3D('',#87409,#61598,#61599) ;
#51959=AXIS2_PLACEMENT_3D('',#87410,#61600,#61601) ;
#51960=AXIS2_PLACEMENT_3D('',#87419,#61606,#61607) ;
#51961=AXIS2_PLACEMENT_3D('',#87422,#61610,#61611) ;
#51962=AXIS2_PLACEMENT_3D('',#87424,#61613,#61614) ;
#51963=AXIS2_PLACEMENT_3D('',#87426,#61616,#61617) ;
#51964=AXIS2_PLACEMENT_3D('',#87428,#61619,#61620) ;
#51965=AXIS2_PLACEMENT_3D('',#87430,#61622,#61623) ;
#51966=AXIS2_PLACEMENT_3D('',#87431,#61624,#61625) ;
#51967=AXIS2_PLACEMENT_3D('',#87433,#61627,#61628) ;
#51968=AXIS2_PLACEMENT_3D('',#87434,#61629,#61630) ;
#51969=AXIS2_PLACEMENT_3D('',#87436,#61632,#61633) ;
#51970=AXIS2_PLACEMENT_3D('',#87438,#61635,#61636) ;
#51971=AXIS2_PLACEMENT_3D('',#87440,#61638,#61639) ;
#51972=AXIS2_PLACEMENT_3D('',#87442,#61641,#61642) ;
#51973=AXIS2_PLACEMENT_3D('',#87444,#61644,#61645) ;
#61018=DIRECTION('axis',(0.,0.,1.)) ;
#61019=DIRECTION('refdir',(1.,0.,0.)) ;
#61020=DIRECTION('center_axis',(-1.,0.,-2.52374105052742E-18)) ;
#61021=DIRECTION('ref_axis',(-1.78455441078632E-18,-0.707106781186736,0.707106781186359)) ;
#61022=DIRECTION('',(1.,0.,2.52374105052742E-18)) ;
#61023=DIRECTION('center_axis',(-1.,0.,0.)) ;
#61024=DIRECTION('ref_axis',(0.,-1.,0.)) ;
#61025=DIRECTION('',(-1.,0.,-2.52374105052742E-18)) ;
#61026=DIRECTION('center_axis',(0.,0.,-1.)) ;
#61027=DIRECTION('ref_axis',(0.707106781186359,-0.707106781186736,0.)) ;
#61028=DIRECTION('center_axis',(0.,0.,-1.)) ;
#61029=DIRECTION('ref_axis',(1.,0.,0.)) ;
#61030=DIRECTION('',(0.,0.,-1.)) ;
#61031=DIRECTION('center_axis',(0.,0.,1.)) ;
#61032=DIRECTION('ref_axis',(0.,-1.,0.)) ;
#61033=DIRECTION('',(0.,0.,1.)) ;
#61034=DIRECTION('center_axis',(-1.,0.,-2.52374105052742E-18)) ;
#61035=DIRECTION('ref_axis',(1.78455441078632E-18,-0.707106781186736,-0.707106781186359)) ;
#61036=DIRECTION('',(1.,0.,2.52374105052742E-18)) ;
#61037=DIRECTION('center_axis',(-1.,0.,0.)) ;
#61038=DIRECTION('ref_axis',(0.,0.,-1.)) ;
#61039=DIRECTION('',(-1.,0.,-2.52374105052742E-18)) ;
#61040=DIRECTION('center_axis',(-0.81649658092775,-0.408248290463875,-0.408248290463804)) ;
#61041=DIRECTION('ref_axis',(0.57735026918959,-0.577350269189732,-0.577350269189555)) ;
#61042=DIRECTION('center_axis',(3.36764187079272E-15,-1.,7.93867294829711E-33)) ;
#61043=DIRECTION('ref_axis',(0.707106781186547,2.38128240344528E-15,-0.707106781186547)) ;
#61044=DIRECTION('center_axis',(-0.81649658092775,-0.408248290463875,0.408248290463804)) ;
#61045=DIRECTION('ref_axis',(0.577350269189602,-0.577350269189744,0.577350269189531)) ;
#61046=DIRECTION('center_axis',(3.36764187079272E-15,-1.,7.93867294829711E-33)) ;
#61047=DIRECTION('ref_axis',(0.707106781186547,2.38128240344528E-15,0.707106781186547)) ;
#61048=DIRECTION('center_axis',(2.52374105052742E-18,5.60383084497445E-34,
-1.)) ;
#61049=DIRECTION('ref_axis',(1.,3.40207761657885E-68,2.52374105052742E-18)) ;
#61050=DIRECTION('',(3.36764187079272E-15,-1.,7.93867294829711E-33)) ;
#61051=DIRECTION('center_axis',(-2.52374105052742E-18,-5.60383084497445E-34,
1.)) ;
#61052=DIRECTION('ref_axis',(-0.707106781186548,0.707106781186548,-1.7845544107868E-18)) ;
#61053=DIRECTION('',(1.41426179436738E-51,-1.,-5.60383084497445E-34)) ;
#61054=DIRECTION('',(-1.,0.,-2.52374105052742E-18)) ;
#61055=DIRECTION('',(-0.212265141871518,-0.977212110826644,-5.35702252137179E-19)) ;
#61056=DIRECTION('',(1.41426179436738E-51,-1.,-5.60383084497445E-34)) ;
#61057=DIRECTION('',(-1.,0.,-2.52374105052742E-18)) ;
#61058=DIRECTION('center_axis',(2.52374105052742E-18,5.60383084497445E-34,
-1.)) ;
#61059=DIRECTION('ref_axis',(0.422618261740848,-0.906307787036581,1.06657905585792E-18)) ;
#61060=DIRECTION('',(-0.642787609686526,-0.766044443118989,-1.62222947733628E-18)) ;
#61061=DIRECTION('center_axis',(2.52374105052742E-18,5.60383084497445E-34,
-1.)) ;
#61062=DIRECTION('ref_axis',(0.939692620785894,-0.342020143325708,2.37154084195506E-18)) ;
#61063=DIRECTION('',(-1.0449157878825E-14,-1.,-2.69313517667302E-32)) ;
#61064=DIRECTION('center_axis',(2.52374105052742E-18,5.60383084497445E-34,
-1.)) ;
#61065=DIRECTION('ref_axis',(0.939692620785894,0.342020143325708,2.37154084195506E-18)) ;
#61066=DIRECTION('',(0.642787609686559,-0.766044443118961,1.62222947733637E-18)) ;
#61067=DIRECTION('center_axis',(2.52374105052742E-18,5.60383084497445E-34,
-1.)) ;
#61068=DIRECTION('ref_axis',(0.422618261740652,0.906307787036672,1.06657905585743E-18)) ;
#61069=DIRECTION('',(1.,0.,2.52374105052742E-18)) ;
#61070=DIRECTION('',(1.41426179436738E-51,-1.,-5.60383084497445E-34)) ;
#61071=DIRECTION('',(1.,-5.00382208281761E-15,2.52374105052742E-18)) ;
#61072=DIRECTION('',(1.41426179436738E-51,-1.,-5.60383084497445E-34)) ;
#61073=DIRECTION('',(1.,0.,2.52374105052742E-18)) ;
#61074=DIRECTION('',(7.65671051465623E-16,1.,2.49273854828173E-33)) ;
#61075=DIRECTION('',(-1.,0.,-2.52374105052742E-18)) ;
#61076=DIRECTION('',(-1.41426179436738E-51,1.,5.60383084497445E-34)) ;
#61077=DIRECTION('',(0.445803505996966,-0.895130847441207,1.12509260855359E-18)) ;
#61078=DIRECTION('center_axis',(2.52374105052742E-18,5.60383084497445E-34,
-1.)) ;
#61079=DIRECTION('ref_axis',(1.,-1.41426179436738E-51,2.52374105052742E-18)) ;
#61080=DIRECTION('',(1.41426179436738E-51,-1.,-5.60383084497445E-34)) ;
#61081=DIRECTION('center_axis',(-2.52374105052742E-18,-5.60383084497445E-34,
1.)) ;
#61082=DIRECTION('ref_axis',(1.73732004304105E-19,1.,5.60821539088498E-34)) ;
#61083=DIRECTION('',(-1.41426179436738E-51,1.,5.60383084497445E-34)) ;
#61084=DIRECTION('center_axis',(-2.52374105052742E-18,-5.60383084497445E-34,
1.)) ;
#61085=DIRECTION('ref_axis',(1.73732004304105E-19,-1.,-5.59944629906392E-34)) ;
#61086=DIRECTION('',(1.,0.,2.52374105052742E-18)) ;
#61087=DIRECTION('',(1.41426179436738E-51,-1.,-5.60383084497445E-34)) ;
#61088=DIRECTION('',(-1.,0.,-2.52374105052742E-18)) ;
#61089=DIRECTION('',(-1.41426179436738E-51,1.,5.60383084497445E-34)) ;
#61090=DIRECTION('',(-1.,0.,-2.52374105052742E-18)) ;
#61091=DIRECTION('',(-1.41426179436738E-51,1.,5.60383084497445E-34)) ;
#61092=DIRECTION('',(1.,0.,2.52374105052742E-18)) ;
#61093=DIRECTION('',(1.41426179436738E-51,-1.,-5.60383084497445E-34)) ;
#61094=DIRECTION('',(-1.,0.,-2.52374105052742E-18)) ;
#61095=DIRECTION('',(-1.41426179436738E-51,1.,5.60383084497445E-34)) ;
#61096=DIRECTION('',(1.,0.,2.52374105052742E-18)) ;
#61097=DIRECTION('',(1.41426179436738E-51,-1.,-5.60383084497445E-34)) ;
#61098=DIRECTION('',(-1.,0.,-2.52374105052742E-18)) ;
#61099=DIRECTION('',(-1.41426179436738E-51,1.,5.60383084497445E-34)) ;
#61100=DIRECTION('',(1.,0.,2.52374105052742E-18)) ;
#61101=DIRECTION('',(1.41426179436738E-51,-1.,-5.60383084497445E-34)) ;
#61102=DIRECTION('center_axis',(3.36764187079272E-15,-1.,7.93867294829711E-33)) ;
#61103=DIRECTION('ref_axis',(0.707106781186548,2.38128240344528E-15,0.707106781186548)) ;
#61104=DIRECTION('',(-3.36764187079272E-15,1.,-7.93867294829711E-33)) ;
#61105=DIRECTION('center_axis',(0.,1.,0.)) ;
#61106=DIRECTION('ref_axis',(0.,0.,1.)) ;
#61107=DIRECTION('center_axis',(1.,3.36764187079272E-15,0.)) ;
#61108=DIRECTION('ref_axis',(3.36764187079272E-15,-1.,7.93867294829711E-33)) ;
#61109=DIRECTION('',(3.36764187079272E-15,-1.,7.93867294829711E-33)) ;
#61110=DIRECTION('',(0.,0.,-1.)) ;
#61111=DIRECTION('center_axis',(3.36764187079272E-15,-1.,7.93867294829711E-33)) ;
#61112=DIRECTION('ref_axis',(0.707106781186548,2.38128240344528E-15,-0.707106781186548)) ;
#61113=DIRECTION('',(-3.36764187079272E-15,1.,-7.93867294829711E-33)) ;
#61114=DIRECTION('center_axis',(0.,1.,0.)) ;
#61115=DIRECTION('ref_axis',(1.,0.,0.)) ;
#61116=DIRECTION('center_axis',(2.52374105052742E-18,5.60383084497445E-34,
-1.)) ;
#61117=DIRECTION('ref_axis',(1.,3.40207761657885E-68,2.52374105052742E-18)) ;
#61118=DIRECTION('center_axis',(-2.52374105052742E-18,-5.60383084497445E-34,
1.)) ;
#61119=DIRECTION('ref_axis',(1.,-1.41426179436738E-51,2.52374105052742E-18)) ;
#61120=DIRECTION('',(-0.445803505996966,0.895130847441207,-1.12509260855359E-18)) ;
#61121=DIRECTION('',(-1.41426179436738E-51,1.,5.60383084497445E-34)) ;
#61122=DIRECTION('',(-1.,0.,-2.52374105052742E-18)) ;
#61123=DIRECTION('',(7.65671051465623E-16,1.,2.49273854828173E-33)) ;
#61124=DIRECTION('',(1.,0.,2.52374105052742E-18)) ;
#61125=DIRECTION('',(1.41426179436738E-51,-1.,-5.60383084497445E-34)) ;
#61126=DIRECTION('',(1.,-5.00382208281761E-15,2.52374105052742E-18)) ;
#61127=DIRECTION('',(-1.41426179436738E-51,1.,5.60383084497445E-34)) ;
#61128=DIRECTION('',(-1.,0.,-2.52374105052742E-18)) ;
#61129=DIRECTION('center_axis',(-2.52374105052742E-18,-5.60383084497445E-34,
1.)) ;
#61130=DIRECTION('ref_axis',(0.422618261740652,0.906307787036672,1.06657905585743E-18)) ;
#61131=DIRECTION('',(-0.642787609686559,0.766044443118961,-1.62222947733637E-18)) ;
#61132=DIRECTION('center_axis',(-2.52374105052742E-18,-5.60383084497445E-34,
1.)) ;
#61133=DIRECTION('ref_axis',(0.939692620785894,0.342020143325708,2.37154084195506E-18)) ;
#61134=DIRECTION('',(1.0449157878825E-14,1.,2.69313517667302E-32)) ;
#61135=DIRECTION('center_axis',(-2.52374105052742E-18,-5.60383084497445E-34,
1.)) ;
#61136=DIRECTION('ref_axis',(0.939692620785894,-0.342020143325708,2.37154084195506E-18)) ;
#61137=DIRECTION('',(0.642787609686526,0.766044443118989,1.62222947733628E-18)) ;
#61138=DIRECTION('center_axis',(-2.52374105052742E-18,-5.60383084497445E-34,
1.)) ;
#61139=DIRECTION('ref_axis',(0.422618261740848,-0.906307787036581,1.06657905585792E-18)) ;
#61140=DIRECTION('',(1.,0.,2.52374105052742E-18)) ;
#61141=DIRECTION('',(-1.41426179436738E-51,1.,5.60383084497445E-34)) ;
#61142=DIRECTION('',(0.212265141871518,0.977212110826644,5.35702252137179E-19)) ;
#61143=DIRECTION('',(-1.,0.,-2.52374105052742E-18)) ;
#61144=DIRECTION('',(1.41426179436738E-51,-1.,-5.60383084497445E-34)) ;
#61145=DIRECTION('center_axis',(2.52374105052742E-18,5.60383084497445E-34,
-1.)) ;
#61146=DIRECTION('ref_axis',(-0.707106781186548,0.707106781186548,-1.7845544107868E-18)) ;
#61147=DIRECTION('center_axis',(-2.52374105052742E-18,-5.60383084497445E-34,
1.)) ;
#61148=DIRECTION('ref_axis',(-1.,-3.40207761657885E-68,-2.52374105052742E-18)) ;
#61149=DIRECTION('',(1.41426179436738E-51,-1.,-5.60383084497445E-34)) ;
#61150=DIRECTION('center_axis',(-2.52374105052742E-18,-5.60383084497445E-34,
1.)) ;
#61151=DIRECTION('ref_axis',(1.,3.40207761657885E-68,2.52374105052742E-18)) ;
#61152=DIRECTION('',(-1.41426179436738E-51,1.,5.60383084497445E-34)) ;
#61153=DIRECTION('',(-1.41426179436738E-51,1.,5.60383084497445E-34)) ;
#61154=DIRECTION('',(-1.,0.,-2.52374105052742E-18)) ;
#61155=DIRECTION('',(1.41426179436738E-51,-1.,-5.60383084497445E-34)) ;
#61156=DIRECTION('',(1.,0.,2.52374105052742E-18)) ;
#61157=DIRECTION('center_axis',(1.41426179436738E-51,-1.,-5.60383084497445E-34)) ;
#61158=DIRECTION('ref_axis',(0.707106781186548,3.96250679110377E-34,-0.707106781186548)) ;
#61159=DIRECTION('center_axis',(-5.00382208281761E-15,-1.,0.)) ;
#61160=DIRECTION('ref_axis',(0.707106781186548,-3.53823652661133E-15,-0.707106781186548)) ;
#61161=DIRECTION('',(1.41426179436738E-51,-1.,-5.60383084497445E-34)) ;
#61162=DIRECTION('center_axis',(0.70710678118661,-0.707106781186485,0.)) ;
#61163=DIRECTION('ref_axis',(0.707106781186485,0.70710678118661,-6.13317366673295E-17)) ;
#61164=DIRECTION('center_axis',(-1.41426179436738E-51,1.,5.60383084497445E-34)) ;
#61165=DIRECTION('ref_axis',(0.707106781186548,-3.96250679110377E-34,0.707106781186548)) ;
#61166=DIRECTION('center_axis',(-5.00382208281761E-15,-1.,0.)) ;
#61167=DIRECTION('ref_axis',(0.707106781186548,-3.53823652661133E-15,0.707106781186548)) ;
#61168=DIRECTION('center_axis',(0.70710678118661,-0.707106781186485,0.)) ;
#61169=DIRECTION('ref_axis',(0.707106781186485,0.70710678118661,6.13317366673295E-17)) ;
#61170=DIRECTION('',(-1.41426179436738E-51,1.,5.60383084497445E-34)) ;
#61171=DIRECTION('center_axis',(1.,1.41426179436738E-51,0.)) ;
#61172=DIRECTION('ref_axis',(1.41426179436738E-51,-1.,-5.60383084497445E-34)) ;
#61173=DIRECTION('',(0.,0.,-1.)) ;
#61174=DIRECTION('',(0.,0.,-1.)) ;
#61175=DIRECTION('center_axis',(2.52374105052742E-18,5.60383084497445E-34,
-1.)) ;
#61176=DIRECTION('ref_axis',(-1.,0.,0.)) ;
#61177=DIRECTION('center_axis',(0.,1.,0.)) ;
#61178=DIRECTION('ref_axis',(1.,0.,0.)) ;
#61179=DIRECTION('center_axis',(0.64278760968649,-0.76604444311902,2.28364033349672E-13)) ;
#61180=DIRECTION('ref_axis',(3.55271367880058E-13,6.95559915454618E-29,
-1.)) ;
#61181=DIRECTION('center_axis',(2.52374105052742E-18,5.60383084497445E-34,
-1.)) ;
#61182=DIRECTION('ref_axis',(0.939692620785894,0.342020143325708,2.37154084195506E-18)) ;
#61183=DIRECTION('center_axis',(2.52374105052742E-18,5.60383084497445E-34,
-1.)) ;
#61184=DIRECTION('ref_axis',(-1.,0.,0.)) ;
#61185=DIRECTION('center_axis',(0.,1.,0.)) ;
#61186=DIRECTION('ref_axis',(1.77635683940029E-13,0.,1.)) ;
#61187=DIRECTION('center_axis',(-2.52374105052742E-18,-5.60383084497445E-34,
1.)) ;
#61188=DIRECTION('ref_axis',(0.939692620785894,0.342020143325708,2.37154084195506E-18)) ;
#61189=DIRECTION('center_axis',(0.64278760968649,-0.76604444311902,-2.28364033349672E-13)) ;
#61190=DIRECTION('ref_axis',(0.76604444311902,0.64278760968649,-2.26813531225949E-29)) ;
#61191=DIRECTION('center_axis',(0.,0.,-1.)) ;
#61192=DIRECTION('ref_axis',(0.939692620785895,0.342020143325706,0.)) ;
#61193=DIRECTION('',(0.,0.,-1.)) ;
#61194=DIRECTION('',(0.,0.,1.)) ;
#61195=DIRECTION('center_axis',(1.,-1.0449157878825E-14,0.)) ;
#61196=DIRECTION('ref_axis',(-1.0449157878825E-14,-1.,-2.69313517667302E-32)) ;
#61197=DIRECTION('',(1.0449157878825E-14,1.,2.69313517667302E-32)) ;
#61198=DIRECTION('',(0.,0.,1.)) ;
#61199=DIRECTION('',(-1.0449157878825E-14,-1.,-2.69313517667302E-32)) ;
#61200=DIRECTION('center_axis',(-1.0449157878825E-14,-1.,-2.69313517667302E-32)) ;
#61201=DIRECTION('ref_axis',(0.707106781186485,-7.38867039380535E-15,0.70710678118661)) ;
#61202=DIRECTION('center_axis',(0.,-1.,0.)) ;
#61203=DIRECTION('ref_axis',(1.,0.,0.)) ;
#61204=DIRECTION('center_axis',(0.642787609686559,-0.766044443118961,1.62222947733637E-18)) ;
#61205=DIRECTION('ref_axis',(0.541675220419852,0.454519477672194,0.707106781186336)) ;
#61206=DIRECTION('',(-0.642787609686559,0.766044443118961,-1.62222947733637E-18)) ;
#61207=DIRECTION('center_axis',(-0.64278760968649,0.76604444311902,0.)) ;
#61208=DIRECTION('ref_axis',(0.,0.,1.)) ;
#61209=DIRECTION('center_axis',(2.52374105052742E-18,5.60383084497445E-34,
-1.)) ;
#61210=DIRECTION('ref_axis',(-1.,0.,0.)) ;
#61211=DIRECTION('center_axis',(-0.64278760968649,0.76604444311902,0.)) ;
#61212=DIRECTION('ref_axis',(0.76604444311902,0.64278760968649,0.)) ;
#61213=DIRECTION('center_axis',(1.,0.,0.)) ;
#61214=DIRECTION('ref_axis',(0.,0.,-1.)) ;
#61215=DIRECTION('center_axis',(2.52374105052742E-18,5.60383084497445E-34,
-1.)) ;
#61216=DIRECTION('ref_axis',(0.422618261740652,0.906307787036672,1.06657905585743E-18)) ;
#61217=DIRECTION('center_axis',(2.52374105052742E-18,5.60383084497445E-34,
-1.)) ;
#61218=DIRECTION('ref_axis',(-1.,0.,0.)) ;
#61219=DIRECTION('center_axis',(-2.52374105052742E-18,-5.60383084497445E-34,
1.)) ;
#61220=DIRECTION('ref_axis',(0.422618261740652,0.906307787036672,1.06657905585743E-18)) ;
#61221=DIRECTION('center_axis',(1.,0.,0.)) ;
#61222=DIRECTION('ref_axis',(0.,1.,0.)) ;
#61223=DIRECTION('center_axis',(0.,0.,-1.)) ;
#61224=DIRECTION('ref_axis',(0.422618261740691,0.906307787036654,0.)) ;
#61225=DIRECTION('',(0.,0.,-1.)) ;
#61226=DIRECTION('',(0.,0.,1.)) ;
#61227=DIRECTION('center_axis',(0.642787609686559,-0.766044443118961,1.62222947733637E-18)) ;
#61228=DIRECTION('ref_axis',(0.541675220419655,0.454519477672028,-0.707106781186594)) ;
#61229=DIRECTION('',(0.642787609686559,-0.766044443118961,1.62222947733637E-18)) ;
#61230=DIRECTION('center_axis',(0.766044443118961,0.642787609686559,0.)) ;
#61231=DIRECTION('ref_axis',(0.642787609686559,-0.766044443118961,1.62222947733637E-18)) ;
#61232=DIRECTION('center_axis',(2.52374105052742E-18,5.60383084497445E-34,
-1.)) ;
#61233=DIRECTION('ref_axis',(-1.,0.,0.)) ;
#61234=DIRECTION('center_axis',(0.64278760968649,0.76604444311902,1.14182016674836E-13)) ;
#61235=DIRECTION('ref_axis',(0.76604444311902,-0.64278760968649,1.13406765612974E-29)) ;
#61236=DIRECTION('center_axis',(0.,-1.,0.)) ;
#61237=DIRECTION('ref_axis',(1.77635683940029E-13,0.,-1.)) ;
#61238=DIRECTION('center_axis',(2.52374105052742E-18,5.60383084497445E-34,
-1.)) ;
#61239=DIRECTION('ref_axis',(0.939692620785894,-0.342020143325708,2.37154084195506E-18)) ;
#61240=DIRECTION('center_axis',(2.52374105052742E-18,5.60383084497445E-34,
-1.)) ;
#61241=DIRECTION('ref_axis',(-1.,0.,0.)) ;
#61242=DIRECTION('center_axis',(0.64278760968649,0.76604444311902,-1.14182016674836E-13)) ;
#61243=DIRECTION('ref_axis',(1.77635683940029E-13,-3.47779957727309E-29,
1.)) ;
#61244=DIRECTION('center_axis',(-2.52374105052742E-18,-5.60383084497445E-34,
1.)) ;
#61245=DIRECTION('ref_axis',(0.939692620785894,-0.342020143325708,2.37154084195506E-18)) ;
#61246=DIRECTION('center_axis',(0.,0.,-1.)) ;
#61247=DIRECTION('ref_axis',(0.939692620785895,-0.342020143325706,0.)) ;
#61248=DIRECTION('',(0.,0.,-1.)) ;
#61249=DIRECTION('center_axis',(-0.642787609686526,-0.76604444311899,-1.62222947733628E-18)) ;
#61250=DIRECTION('ref_axis',(0.541675220419675,-0.454519477672004,-0.707106781186594)) ;
#61251=DIRECTION('',(-0.642787609686526,-0.766044443118989,-1.62222947733628E-18)) ;
#61252=DIRECTION('center_axis',(-0.642787609686402,-0.766044443119093,0.)) ;
#61253=DIRECTION('ref_axis',(0.,0.,-1.)) ;
#61254=DIRECTION('center_axis',(0.76604444311899,-0.642787609686526,0.)) ;
#61255=DIRECTION('ref_axis',(-0.642787609686526,-0.766044443118989,-1.62222947733628E-18)) ;
#61256=DIRECTION('',(0.642787609686526,0.766044443118989,1.62222947733628E-18)) ;
#61257=DIRECTION('',(0.,0.,1.)) ;
#61258=DIRECTION('center_axis',(-0.642787609686526,-0.76604444311899,-1.62222947733628E-18)) ;
#61259=DIRECTION('ref_axis',(0.541675220419675,-0.454519477672004,0.707106781186594)) ;
#61260=DIRECTION('center_axis',(-0.642787609686402,-0.766044443119093,0.)) ;
#61261=DIRECTION('ref_axis',(0.766044443119093,-0.642787609686402,0.)) ;
#61262=DIRECTION('center_axis',(0.,0.,-1.)) ;
#61263=DIRECTION('ref_axis',(-1.,0.,0.)) ;
#61264=DIRECTION('center_axis',(-0.316227766016905,-0.948683298050491,0.)) ;
#61265=DIRECTION('ref_axis',(0.948683298050491,-0.316227766016905,0.)) ;
#61266=DIRECTION('center_axis',(-0.316227766016905,-0.948683298050491,0.)) ;
#61267=DIRECTION('ref_axis',(0.948683298050491,-0.316227766016905,0.)) ;
#61268=DIRECTION('center_axis',(0.948683298050519,0.316227766016821,0.)) ;
#61269=DIRECTION('ref_axis',(0.316227766016821,-0.948683298050519,0.)) ;
#61270=DIRECTION('center_axis',(0.948683298050519,0.316227766016821,0.)) ;
#61271=DIRECTION('ref_axis',(0.316227766016821,-0.948683298050519,0.)) ;
#61272=DIRECTION('center_axis',(0.,0.,-1.)) ;
#61273=DIRECTION('ref_axis',(-0.70710678118661,0.707106781186485,0.)) ;
#61274=DIRECTION('',(0.,0.,-1.)) ;
#61275=DIRECTION('center_axis',(0.,0.,-1.)) ;
#61276=DIRECTION('ref_axis',(-1.,0.,0.)) ;
#61277=DIRECTION('',(0.,0.,1.)) ;
#61278=DIRECTION('center_axis',(0.948683298050519,0.316227766016821,0.)) ;
#61279=DIRECTION('ref_axis',(0.316227766016821,-0.948683298050519,0.)) ;
#61280=DIRECTION('center_axis',(0.948683298050519,0.316227766016821,0.)) ;
#61281=DIRECTION('ref_axis',(0.316227766016821,-0.948683298050519,0.)) ;
#61282=DIRECTION('center_axis',(-0.316227766016889,-0.948683298050497,0.)) ;
#61283=DIRECTION('ref_axis',(0.948683298050497,-0.316227766016889,0.)) ;
#61284=DIRECTION('center_axis',(-0.316227766016889,-0.948683298050497,0.)) ;
#61285=DIRECTION('ref_axis',(0.948683298050497,-0.316227766016889,0.)) ;
#61286=DIRECTION('center_axis',(1.,1.41426179436738E-51,0.)) ;
#61287=DIRECTION('ref_axis',(1.41426179436738E-51,-1.,-5.60383084497445E-34)) ;
#61288=DIRECTION('',(-1.41426179436738E-51,1.,5.60383084497445E-34)) ;
#61289=DIRECTION('',(0.,0.,-1.)) ;
#61290=DIRECTION('',(1.41426179436738E-51,-1.,-5.60383084497445E-34)) ;
#61291=DIRECTION('center_axis',(1.41426179436738E-51,-1.,-5.60383084497445E-34)) ;
#61292=DIRECTION('ref_axis',(0.70710678118661,-3.96250679110342E-34,0.707106781186485)) ;
#61293=DIRECTION('center_axis',(0.106742421682839,0.994286706847317,0.)) ;
#61294=DIRECTION('ref_axis',(-0.994286706847317,0.106742421682839,5.24986294729659E-33)) ;
#61295=DIRECTION('center_axis',(-1.,0.,-2.52374105052742E-18)) ;
#61296=DIRECTION('ref_axis',(-1.78455441078632E-18,-0.707106781186736,0.707106781186359)) ;
#61297=DIRECTION('',(1.,0.,2.52374105052742E-18)) ;
#61298=DIRECTION('center_axis',(1.,0.,0.)) ;
#61299=DIRECTION('ref_axis',(0.,3.55271367880058E-13,1.)) ;
#61300=DIRECTION('center_axis',(1.,0.,0.)) ;
#61301=DIRECTION('ref_axis',(0.,-1.,0.)) ;
#61302=DIRECTION('center_axis',(2.52374105052742E-18,5.60383084497445E-34,
-1.)) ;
#61303=DIRECTION('ref_axis',(0.422618261740848,-0.906307787036581,1.06657905585792E-18)) ;
#61304=DIRECTION('center_axis',(-2.52374105052742E-18,-5.60383084497445E-34,
1.)) ;
#61305=DIRECTION('ref_axis',(0.422618261740848,-0.906307787036581,1.06657905585792E-18)) ;
#61306=DIRECTION('center_axis',(0.,0.,-1.)) ;
#61307=DIRECTION('ref_axis',(0.422618261740767,-0.906307787036618,0.)) ;
#61308=DIRECTION('',(0.,0.,-1.)) ;
#61309=DIRECTION('center_axis',(-1.,0.,-2.52374105052742E-18)) ;
#61310=DIRECTION('ref_axis',(1.78455441078632E-18,-0.707106781186736,-0.707106781186359)) ;
#61311=DIRECTION('',(-1.,0.,-2.52374105052742E-18)) ;
#61312=DIRECTION('center_axis',(0.,-1.,0.)) ;
#61313=DIRECTION('ref_axis',(-1.,0.,-2.52374105052742E-18)) ;
#61314=DIRECTION('center_axis',(1.41426179436738E-51,-1.,-5.60383084497445E-34)) ;
#61315=DIRECTION('ref_axis',(0.707106781186548,-3.96250679110377E-34,0.707106781186548)) ;
#61316=DIRECTION('center_axis',(0.,-1.,0.)) ;
#61317=DIRECTION('ref_axis',(1.,0.,0.)) ;
#61318=DIRECTION('center_axis',(0.,1.,0.)) ;
#61319=DIRECTION('ref_axis',(0.,0.,1.)) ;
#61320=DIRECTION('',(-1.41426179436738E-51,1.,5.60383084497445E-34)) ;
#61321=DIRECTION('center_axis',(-2.52374105052742E-18,-5.60383084497445E-34,
1.)) ;
#61322=DIRECTION('ref_axis',(1.,0.,0.)) ;
#61323=DIRECTION('center_axis',(0.,-1.,0.)) ;
#61324=DIRECTION('ref_axis',(0.,0.,1.)) ;
#61325=DIRECTION('center_axis',(2.52374105052742E-18,5.60383084497445E-34,
-1.)) ;
#61326=DIRECTION('ref_axis',(1.73732004304105E-19,-1.,-5.59944629906392E-34)) ;
#61327=DIRECTION('center_axis',(-1.41426179436738E-51,1.,5.60383084497445E-34)) ;
#61328=DIRECTION('ref_axis',(-0.707106781186548,-3.96250679110377E-34,0.707106781186548)) ;
#61329=DIRECTION('center_axis',(0.,-1.,0.)) ;
#61330=DIRECTION('ref_axis',(0.,0.,1.)) ;
#61331=DIRECTION('',(1.41426179436738E-51,-1.,-5.60383084497445E-34)) ;
#61332=DIRECTION('center_axis',(-2.52374105052742E-18,-5.60383084497445E-34,
1.)) ;
#61333=DIRECTION('ref_axis',(1.,0.,0.)) ;
#61334=DIRECTION('center_axis',(2.52374105052742E-18,5.60383084497445E-34,
-1.)) ;
#61335=DIRECTION('ref_axis',(1.73732004304105E-19,1.,5.60821539088498E-34)) ;
#61336=DIRECTION('center_axis',(0.,0.,-1.)) ;
#61337=DIRECTION('ref_axis',(-1.,0.,0.)) ;
#61338=DIRECTION('',(0.,0.,-1.)) ;
#61339=DIRECTION('',(0.,0.,-1.)) ;
#61340=DIRECTION('center_axis',(1.,1.41426179436738E-51,0.)) ;
#61341=DIRECTION('ref_axis',(1.41426179436738E-51,-1.,-5.60383084497445E-34)) ;
#61342=DIRECTION('',(0.,0.,-1.)) ;
#61343=DIRECTION('center_axis',(2.52374105052742E-18,5.60383084497445E-34,
-1.)) ;
#61344=DIRECTION('ref_axis',(-1.,0.,0.)) ;
#61345=DIRECTION('center_axis',(2.52374105052742E-18,5.60383084497445E-34,
-1.)) ;
#61346=DIRECTION('ref_axis',(-0.707106781186547,0.707106781186547,-1.7845544107868E-18)) ;
#61347=DIRECTION('center_axis',(0.,1.,0.)) ;
#61348=DIRECTION('ref_axis',(1.,0.,2.52374105052742E-18)) ;
#61349=DIRECTION('',(0.,0.,-1.)) ;
#61350=DIRECTION('',(0.,0.,-1.)) ;
#61351=DIRECTION('center_axis',(0.,0.,-1.)) ;
#61352=DIRECTION('ref_axis',(-1.,0.,0.)) ;
#61353=DIRECTION('center_axis',(-2.52374105052742E-18,-5.60383084497445E-34,
1.)) ;
#61354=DIRECTION('ref_axis',(-0.707106781186547,0.707106781186547,-1.7845544107868E-18)) ;
#61355=DIRECTION('center_axis',(0.,-1.,0.)) ;
#61356=DIRECTION('ref_axis',(-1.,0.,-2.52374105052742E-18)) ;
#61357=DIRECTION('',(0.,0.,-1.)) ;
#61358=DIRECTION('center_axis',(-2.52374105052742E-18,-5.60383084497445E-34,
1.)) ;
#61359=DIRECTION('ref_axis',(1.,0.,0.)) ;
#61360=DIRECTION('center_axis',(1.,1.41426179436738E-51,0.)) ;
#61361=DIRECTION('ref_axis',(1.41426179436738E-51,-1.,-5.60383084497445E-34)) ;
#61362=DIRECTION('',(0.,0.,-1.)) ;
#61363=DIRECTION('center_axis',(-0.212265141871518,-0.977212110826644,-5.35702252137179E-19)) ;
#61364=DIRECTION('ref_axis',(0.690993310223154,-0.150094121226878,-0.707106781186533)) ;
#61365=DIRECTION('',(-0.212265141871518,-0.977212110826644,-5.35702252137179E-19)) ;
#61366=DIRECTION('center_axis',(0.,1.,0.)) ;
#61367=DIRECTION('ref_axis',(1.,0.,-4.23798197414957E-16)) ;
#61368=DIRECTION('center_axis',(-0.106742421682839,-0.994286706847317,0.)) ;
#61369=DIRECTION('ref_axis',(0.994286706847317,-0.106742421682839,5.01864435613725E-18)) ;
#61370=DIRECTION('center_axis',(1.41426179436738E-51,-1.,-5.60383084497445E-34)) ;
#61371=DIRECTION('ref_axis',(0.70710678118661,3.96250679110342E-34,-0.707106781186485)) ;
#61372=DIRECTION('center_axis',(-1.0449157878825E-14,-1.,-2.69313517667302E-32)) ;
#61373=DIRECTION('ref_axis',(0.707106781186485,-7.38867039380535E-15,-0.70710678118661)) ;
#61374=DIRECTION('center_axis',(1.,0.,2.52374105052742E-18)) ;
#61375=DIRECTION('ref_axis',(1.78455441078632E-18,0.707106781186736,-0.707106781186359)) ;
#61376=DIRECTION('',(1.,0.,2.52374105052742E-18)) ;
#61377=DIRECTION('center_axis',(0.,-1.,0.)) ;
#61378=DIRECTION('ref_axis',(-1.,0.,-2.52374105052742E-18)) ;
#61379=DIRECTION('',(0.,0.,-1.)) ;
#61380=DIRECTION('center_axis',(0.,1.,0.)) ;
#61381=DIRECTION('ref_axis',(1.,0.,4.23798197414957E-16)) ;
#61382=DIRECTION('center_axis',(0.977212110826644,-0.212265141871518,0.)) ;
#61383=DIRECTION('ref_axis',(-0.212265141871518,-0.977212110826644,-5.35702252137179E-19)) ;
#61384=DIRECTION('',(0.212265141871518,0.977212110826644,5.35702252137179E-19)) ;
#61385=DIRECTION('center_axis',(0.,1.,0.)) ;
#61386=DIRECTION('ref_axis',(1.,0.,2.52374105052742E-18)) ;
#61387=DIRECTION('',(-1.,0.,-2.52374105052742E-18)) ;
#61388=DIRECTION('center_axis',(1.,0.,2.52374105052742E-18)) ;
#61389=DIRECTION('ref_axis',(-1.78455441078632E-18,0.707106781186736,0.707106781186359)) ;
#61390=DIRECTION('center_axis',(-0.212265141871518,-0.977212110826644,-5.35702252137179E-19)) ;
#61391=DIRECTION('ref_axis',(0.690993310223154,-0.150094121226878,0.707106781186533)) ;
#61392=DIRECTION('center_axis',(1.,1.41426179436738E-51,0.)) ;
#61393=DIRECTION('ref_axis',(0.,0.,-1.)) ;
#61394=DIRECTION('center_axis',(0.,1.,0.)) ;
#61395=DIRECTION('ref_axis',(-1.,0.,0.)) ;
#61396=DIRECTION('center_axis',(-1.,-1.41426179436738E-51,0.)) ;
#61397=DIRECTION('ref_axis',(-9.57459760970815E-52,0.677003200386319,0.735980072193997)) ;
#61398=DIRECTION('center_axis',(1.,1.41426179436738E-51,0.)) ;
#61399=DIRECTION('ref_axis',(-9.57459760970815E-52,0.677003200386319,0.735980072193997)) ;
#61400=DIRECTION('center_axis',(1.41426179436738E-51,-1.,0.)) ;
#61401=DIRECTION('ref_axis',(-0.707106781186568,-1.00003410517026E-51,0.707106781186527)) ;
#61402=DIRECTION('center_axis',(0.,1.,0.)) ;
#61403=DIRECTION('ref_axis',(-1.,0.,0.)) ;
#61404=DIRECTION('',(-1.41426179436738E-51,1.,0.)) ;
#61405=DIRECTION('',(1.41426179436738E-51,-1.,0.)) ;
#61406=DIRECTION('center_axis',(1.,1.41426179436738E-51,0.)) ;
#61407=DIRECTION('ref_axis',(0.,0.,-1.)) ;
#61408=DIRECTION('center_axis',(-1.,-1.41426179436738E-51,0.)) ;
#61409=DIRECTION('ref_axis',(9.5745976097084E-52,-0.677003200386337,0.735980072193981)) ;
#61410=DIRECTION('center_axis',(1.,1.41426179436738E-51,0.)) ;
#61411=DIRECTION('ref_axis',(9.5745976097084E-52,-0.677003200386337,0.735980072193981)) ;
#61412=DIRECTION('center_axis',(-1.,-1.41426179436738E-51,0.)) ;
#61413=DIRECTION('ref_axis',(1.41426179436738E-51,-1.,-5.60383084497445E-34)) ;
#61414=DIRECTION('center_axis',(-1.,-1.41426179436738E-51,0.)) ;
#61415=DIRECTION('ref_axis',(0.,0.,1.)) ;
#61416=DIRECTION('center_axis',(0.,-1.,0.)) ;
#61417=DIRECTION('ref_axis',(1.,0.,0.)) ;
#61418=DIRECTION('center_axis',(1.,1.41426179436738E-51,0.)) ;
#61419=DIRECTION('ref_axis',(9.5745976097084E-52,-0.677003200386337,0.735980072193981)) ;
#61420=DIRECTION('center_axis',(-1.,-1.41426179436738E-51,0.)) ;
#61421=DIRECTION('ref_axis',(9.5745976097084E-52,-0.677003200386337,0.735980072193981)) ;
#61422=DIRECTION('center_axis',(-1.41426179436738E-51,1.,0.)) ;
#61423=DIRECTION('ref_axis',(0.707106781186568,1.00003410517026E-51,0.707106781186527)) ;
#61424=DIRECTION('center_axis',(0.,-1.,0.)) ;
#61425=DIRECTION('ref_axis',(1.,0.,0.)) ;
#61426=DIRECTION('',(1.41426179436738E-51,-1.,0.)) ;
#61427=DIRECTION('',(-1.41426179436738E-51,1.,0.)) ;
#61428=DIRECTION('center_axis',(-1.,-1.41426179436738E-51,0.)) ;
#61429=DIRECTION('ref_axis',(0.,0.,1.)) ;
#61430=DIRECTION('center_axis',(1.,1.41426179436738E-51,0.)) ;
#61431=DIRECTION('ref_axis',(-9.57459760970815E-52,0.677003200386319,0.735980072193997)) ;
#61432=DIRECTION('center_axis',(-1.,-1.41426179436738E-51,0.)) ;
#61433=DIRECTION('ref_axis',(-9.57459760970815E-52,0.677003200386319,0.735980072193997)) ;
#61434=DIRECTION('center_axis',(1.,1.41426179436738E-51,0.)) ;
#61435=DIRECTION('ref_axis',(-1.41426179436738E-51,1.,5.60383084497445E-34)) ;
#61436=DIRECTION('center_axis',(-1.,-1.41426179436738E-51,0.)) ;
#61437=DIRECTION('ref_axis',(0.,0.,1.)) ;
#61438=DIRECTION('center_axis',(0.,-1.,0.)) ;
#61439=DIRECTION('ref_axis',(1.,0.,0.)) ;
#61440=DIRECTION('center_axis',(1.,1.41426179436738E-51,0.)) ;
#61441=DIRECTION('ref_axis',(9.57459760970815E-52,-0.677003200386319,0.735980072193997)) ;
#61442=DIRECTION('center_axis',(-1.,-1.41426179436738E-51,0.)) ;
#61443=DIRECTION('ref_axis',(9.57459760970815E-52,-0.677003200386319,0.735980072193997)) ;
#61444=DIRECTION('center_axis',(-1.41426179436738E-51,1.,0.)) ;
#61445=DIRECTION('ref_axis',(0.707106781186547,1.00003410517023E-51,0.707106781186547)) ;
#61446=DIRECTION('center_axis',(0.,-1.,0.)) ;
#61447=DIRECTION('ref_axis',(1.,0.,0.)) ;
#61448=DIRECTION('',(1.41426179436738E-51,-1.,0.)) ;
#61449=DIRECTION('',(-1.41426179436738E-51,1.,0.)) ;
#61450=DIRECTION('center_axis',(-1.,-1.41426179436738E-51,0.)) ;
#61451=DIRECTION('ref_axis',(0.,0.,1.)) ;
#61452=DIRECTION('center_axis',(1.,1.41426179436738E-51,0.)) ;
#61453=DIRECTION('ref_axis',(-9.57459760970815E-52,0.677003200386319,0.735980072193997)) ;
#61454=DIRECTION('center_axis',(-1.,-1.41426179436738E-51,0.)) ;
#61455=DIRECTION('ref_axis',(-9.57459760970815E-52,0.677003200386319,0.735980072193997)) ;
#61456=DIRECTION('center_axis',(1.,1.41426179436738E-51,0.)) ;
#61457=DIRECTION('ref_axis',(-1.41426179436738E-51,1.,5.60383084497445E-34)) ;
#61458=DIRECTION('center_axis',(1.,1.41426179436738E-51,0.)) ;
#61459=DIRECTION('ref_axis',(0.,0.,-1.)) ;
#61460=DIRECTION('center_axis',(0.,1.,0.)) ;
#61461=DIRECTION('ref_axis',(-1.,0.,0.)) ;
#61462=DIRECTION('center_axis',(-1.,-1.41426179436738E-51,0.)) ;
#61463=DIRECTION('ref_axis',(-9.57459760970815E-52,0.677003200386319,0.735980072193997)) ;
#61464=DIRECTION('center_axis',(1.,1.41426179436738E-51,0.)) ;
#61465=DIRECTION('ref_axis',(-9.57459760970815E-52,0.677003200386319,0.735980072193997)) ;
#61466=DIRECTION('center_axis',(1.41426179436738E-51,-1.,0.)) ;
#61467=DIRECTION('ref_axis',(-0.707106781186547,-1.00003410517023E-51,0.707106781186547)) ;
#61468=DIRECTION('center_axis',(0.,1.,0.)) ;
#61469=DIRECTION('ref_axis',(-1.,0.,0.)) ;
#61470=DIRECTION('',(-1.41426179436738E-51,1.,0.)) ;
#61471=DIRECTION('',(1.41426179436738E-51,-1.,0.)) ;
#61472=DIRECTION('center_axis',(1.,1.41426179436738E-51,0.)) ;
#61473=DIRECTION('ref_axis',(0.,0.,-1.)) ;
#61474=DIRECTION('center_axis',(-1.,-1.41426179436738E-51,0.)) ;
#61475=DIRECTION('ref_axis',(9.57459760970815E-52,-0.677003200386319,0.735980072193997)) ;
#61476=DIRECTION('center_axis',(1.,1.41426179436738E-51,0.)) ;
#61477=DIRECTION('ref_axis',(9.57459760970815E-52,-0.677003200386319,0.735980072193997)) ;
#61478=DIRECTION('center_axis',(-1.,-1.41426179436738E-51,0.)) ;
#61479=DIRECTION('ref_axis',(1.41426179436738E-51,-1.,-5.60383084497445E-34)) ;
#61480=DIRECTION('center_axis',(-1.,-1.41426179436738E-51,0.)) ;
#61481=DIRECTION('ref_axis',(0.,0.,1.)) ;
#61482=DIRECTION('center_axis',(0.,-1.,0.)) ;
#61483=DIRECTION('ref_axis',(1.,0.,0.)) ;
#61484=DIRECTION('center_axis',(1.,1.41426179436738E-51,0.)) ;
#61485=DIRECTION('ref_axis',(9.57459760970815E-52,-0.677003200386319,0.735980072193997)) ;
#61486=DIRECTION('center_axis',(-1.,-1.41426179436738E-51,0.)) ;
#61487=DIRECTION('ref_axis',(9.57459760970815E-52,-0.677003200386319,0.735980072193997)) ;
#61488=DIRECTION('center_axis',(-1.41426179436738E-51,1.,0.)) ;
#61489=DIRECTION('ref_axis',(0.707106781186568,1.00003410517026E-51,0.707106781186527)) ;
#61490=DIRECTION('center_axis',(0.,-1.,0.)) ;
#61491=DIRECTION('ref_axis',(1.,0.,0.)) ;
#61492=DIRECTION('',(1.41426179436738E-51,-1.,0.)) ;
#61493=DIRECTION('',(-1.41426179436738E-51,1.,0.)) ;
#61494=DIRECTION('center_axis',(-1.,-1.41426179436738E-51,0.)) ;
#61495=DIRECTION('ref_axis',(0.,0.,1.)) ;
#61496=DIRECTION('center_axis',(1.,1.41426179436738E-51,0.)) ;
#61497=DIRECTION('ref_axis',(-9.5745976097084E-52,0.677003200386337,0.735980072193981)) ;
#61498=DIRECTION('center_axis',(-1.,-1.41426179436738E-51,0.)) ;
#61499=DIRECTION('ref_axis',(-9.5745976097084E-52,0.677003200386337,0.735980072193981)) ;
#61500=DIRECTION('center_axis',(1.,1.41426179436738E-51,0.)) ;
#61501=DIRECTION('ref_axis',(-1.41426179436738E-51,1.,5.60383084497445E-34)) ;
#61502=DIRECTION('center_axis',(1.,1.41426179436738E-51,0.)) ;
#61503=DIRECTION('ref_axis',(0.,0.,-1.)) ;
#61504=DIRECTION('center_axis',(0.,1.,0.)) ;
#61505=DIRECTION('ref_axis',(-1.,0.,0.)) ;
#61506=DIRECTION('center_axis',(-1.,-1.41426179436738E-51,0.)) ;
#61507=DIRECTION('ref_axis',(-9.5745976097084E-52,0.677003200386337,0.735980072193981)) ;
#61508=DIRECTION('center_axis',(1.,1.41426179436738E-51,0.)) ;
#61509=DIRECTION('ref_axis',(-9.5745976097084E-52,0.677003200386337,0.735980072193981)) ;
#61510=DIRECTION('center_axis',(1.41426179436738E-51,-1.,0.)) ;
#61511=DIRECTION('ref_axis',(-0.707106781186568,-1.00003410517026E-51,0.707106781186527)) ;
#61512=DIRECTION('center_axis',(0.,1.,0.)) ;
#61513=DIRECTION('ref_axis',(-1.,0.,0.)) ;
#61514=DIRECTION('',(-1.41426179436738E-51,1.,0.)) ;
#61515=DIRECTION('',(1.41426179436738E-51,-1.,0.)) ;
#61516=DIRECTION('center_axis',(1.,1.41426179436738E-51,0.)) ;
#61517=DIRECTION('ref_axis',(0.,0.,-1.)) ;
#61518=DIRECTION('center_axis',(-1.,-1.41426179436738E-51,0.)) ;
#61519=DIRECTION('ref_axis',(9.57459760970815E-52,-0.677003200386319,0.735980072193997)) ;
#61520=DIRECTION('center_axis',(1.,1.41426179436738E-51,0.)) ;
#61521=DIRECTION('ref_axis',(9.57459760970815E-52,-0.677003200386319,0.735980072193997)) ;
#61522=DIRECTION('center_axis',(-1.,-1.41426179436738E-51,0.)) ;
#61523=DIRECTION('ref_axis',(1.41426179436738E-51,-1.,-5.60383084497445E-34)) ;
#61524=DIRECTION('center_axis',(-1.,-1.41426179436738E-51,0.)) ;
#61525=DIRECTION('ref_axis',(0.,0.,1.)) ;
#61526=DIRECTION('center_axis',(0.,-1.,0.)) ;
#61527=DIRECTION('ref_axis',(1.,0.,0.)) ;
#61528=DIRECTION('center_axis',(1.,1.41426179436738E-51,0.)) ;
#61529=DIRECTION('ref_axis',(9.57459760970817E-52,-0.677003200386321,0.735980072193996)) ;
#61530=DIRECTION('center_axis',(-1.,-1.41426179436738E-51,0.)) ;
#61531=DIRECTION('ref_axis',(9.57459760970817E-52,-0.677003200386321,0.735980072193996)) ;
#61532=DIRECTION('center_axis',(-1.41426179436738E-51,1.,0.)) ;
#61533=DIRECTION('ref_axis',(0.707106781186568,1.00003410517026E-51,0.707106781186527)) ;
#61534=DIRECTION('center_axis',(0.,-1.,0.)) ;
#61535=DIRECTION('ref_axis',(1.,0.,0.)) ;
#61536=DIRECTION('',(1.41426179436738E-51,-1.,0.)) ;
#61537=DIRECTION('',(-1.41426179436738E-51,1.,0.)) ;
#61538=DIRECTION('center_axis',(-1.,-1.41426179436738E-51,0.)) ;
#61539=DIRECTION('ref_axis',(0.,0.,1.)) ;
#61540=DIRECTION('center_axis',(1.,1.41426179436738E-51,0.)) ;
#61541=DIRECTION('ref_axis',(-9.57459760970815E-52,0.677003200386319,0.735980072193997)) ;
#61542=DIRECTION('center_axis',(-1.,-1.41426179436738E-51,0.)) ;
#61543=DIRECTION('ref_axis',(-9.57459760970815E-52,0.677003200386319,0.735980072193997)) ;
#61544=DIRECTION('center_axis',(1.,1.41426179436738E-51,0.)) ;
#61545=DIRECTION('ref_axis',(-1.41426179436738E-51,1.,5.60383084497445E-34)) ;
#61546=DIRECTION('center_axis',(1.,1.41426179436738E-51,0.)) ;
#61547=DIRECTION('ref_axis',(0.,0.,-1.)) ;
#61548=DIRECTION('center_axis',(0.,1.,0.)) ;
#61549=DIRECTION('ref_axis',(-1.,0.,0.)) ;
#61550=DIRECTION('center_axis',(-1.,-1.41426179436738E-51,0.)) ;
#61551=DIRECTION('ref_axis',(-9.57459760970817E-52,0.677003200386321,0.735980072193996)) ;
#61552=DIRECTION('center_axis',(1.,1.41426179436738E-51,0.)) ;
#61553=DIRECTION('ref_axis',(-9.57459760970817E-52,0.677003200386321,0.735980072193996)) ;
#61554=DIRECTION('center_axis',(1.41426179436738E-51,-1.,0.)) ;
#61555=DIRECTION('ref_axis',(-0.707106781186568,-1.00003410517026E-51,0.707106781186527)) ;
#61556=DIRECTION('center_axis',(0.,1.,0.)) ;
#61557=DIRECTION('ref_axis',(-1.,0.,0.)) ;
#61558=DIRECTION('',(-1.41426179436738E-51,1.,0.)) ;
#61559=DIRECTION('',(1.41426179436738E-51,-1.,0.)) ;
#61560=DIRECTION('center_axis',(1.,1.41426179436738E-51,0.)) ;
#61561=DIRECTION('ref_axis',(0.,0.,-1.)) ;
#61562=DIRECTION('center_axis',(-1.,-1.41426179436738E-51,0.)) ;
#61563=DIRECTION('ref_axis',(9.57459760970815E-52,-0.677003200386319,0.735980072193997)) ;
#61564=DIRECTION('center_axis',(1.,1.41426179436738E-51,0.)) ;
#61565=DIRECTION('ref_axis',(9.57459760970815E-52,-0.677003200386319,0.735980072193997)) ;
#61566=DIRECTION('center_axis',(-1.,-1.41426179436738E-51,0.)) ;
#61567=DIRECTION('ref_axis',(1.41426179436738E-51,-1.,-5.60383084497445E-34)) ;
#61568=DIRECTION('center_axis',(1.,0.,0.)) ;
#61569=DIRECTION('ref_axis',(0.,0.996521728591783,0.083333333333332)) ;
#61570=DIRECTION('',(1.,0.,0.)) ;
#61571=DIRECTION('center_axis',(0.,0.,1.)) ;
#61572=DIRECTION('ref_axis',(1.,0.,0.)) ;
#61573=DIRECTION('',(-1.,0.,0.)) ;
#61574=DIRECTION('center_axis',(-1.,0.,0.)) ;
#61575=DIRECTION('ref_axis',(0.,-0.996521728591783,0.083333333333332)) ;
#61576=DIRECTION('center_axis',(1.,0.,0.)) ;
#61577=DIRECTION('ref_axis',(0.,0.996521728591783,0.083333333333332)) ;
#61578=DIRECTION('',(1.,0.,0.)) ;
#61579=DIRECTION('center_axis',(0.,0.,1.)) ;
#61580=DIRECTION('ref_axis',(1.,0.,0.)) ;
#61581=DIRECTION('',(-1.,0.,0.)) ;
#61582=DIRECTION('center_axis',(-1.,0.,0.)) ;
#61583=DIRECTION('ref_axis',(0.,-0.996521728591783,0.083333333333332)) ;
#61584=DIRECTION('center_axis',(-1.,0.,0.)) ;
#61585=DIRECTION('ref_axis',(0.,-0.996521728591783,0.083333333333332)) ;
#61586=DIRECTION('',(-1.,0.,0.)) ;
#61587=DIRECTION('center_axis',(0.,0.,1.)) ;
#61588=DIRECTION('ref_axis',(1.,0.,0.)) ;
#61589=DIRECTION('',(1.,0.,0.)) ;
#61590=DIRECTION('center_axis',(1.,0.,0.)) ;
#61591=DIRECTION('ref_axis',(0.,0.996521728591783,0.083333333333332)) ;
#61592=DIRECTION('center_axis',(1.,0.,0.)) ;
#61593=DIRECTION('ref_axis',(0.,0.996521728591783,0.083333333333332)) ;
#61594=DIRECTION('',(1.,0.,0.)) ;
#61595=DIRECTION('center_axis',(0.,0.,1.)) ;
#61596=DIRECTION('ref_axis',(1.,0.,0.)) ;
#61597=DIRECTION('',(-1.,0.,0.)) ;
#61598=DIRECTION('center_axis',(-1.,0.,0.)) ;
#61599=DIRECTION('ref_axis',(0.,-0.996521728591783,0.083333333333332)) ;
#61600=DIRECTION('center_axis',(2.52374105052742E-18,5.60383084497445E-34,
-1.)) ;
#61601=DIRECTION('ref_axis',(1.,3.40207761657885E-68,2.52374105052742E-18)) ;
#61602=DIRECTION('',(-1.41426179436738E-51,1.,5.60383084497445E-34)) ;
#61603=DIRECTION('',(1.,0.,2.52374105052742E-18)) ;
#61604=DIRECTION('',(1.41426179436738E-51,-1.,-5.60383084497445E-34)) ;
#61605=DIRECTION('',(-1.,0.,-2.52374105052742E-18)) ;
#61606=DIRECTION('center_axis',(0.,-1.,0.)) ;
#61607=DIRECTION('ref_axis',(-1.,0.,-2.52374105052742E-18)) ;
#61608=DIRECTION('',(0.,0.,-1.)) ;
#61609=DIRECTION('',(0.,0.,-1.)) ;
#61610=DIRECTION('center_axis',(1.,1.41426179436738E-51,0.)) ;
#61611=DIRECTION('ref_axis',(1.41426179436738E-51,-1.,-5.60383084497445E-34)) ;
#61612=DIRECTION('',(0.,0.,-1.)) ;
#61613=DIRECTION('center_axis',(0.,0.,-1.)) ;
#61614=DIRECTION('ref_axis',(1.,0.,0.)) ;
#61615=DIRECTION('',(0.,0.,1.)) ;
#61616=DIRECTION('center_axis',(-0.895130847441207,-0.445803505996966,0.)) ;
#61617=DIRECTION('ref_axis',(-0.445803505996966,0.895130847441207,-1.12509260855359E-18)) ;
#61618=DIRECTION('',(0.,0.,-1.)) ;
#61619=DIRECTION('center_axis',(-1.,-1.41426179436738E-51,0.)) ;
#61620=DIRECTION('ref_axis',(-1.41426179436738E-51,1.,5.60383084497445E-34)) ;
#61621=DIRECTION('',(0.,0.,-1.)) ;
#61622=DIRECTION('center_axis',(0.,0.,-1.)) ;
#61623=DIRECTION('ref_axis',(1.,0.,0.)) ;
#61624=DIRECTION('center_axis',(0.,1.,0.)) ;
#61625=DIRECTION('ref_axis',(1.,0.,2.52374105052742E-18)) ;
#61626=DIRECTION('',(0.,0.,-1.)) ;
#61627=DIRECTION('center_axis',(-1.,-1.41426179436738E-51,0.)) ;
#61628=DIRECTION('ref_axis',(-1.41426179436738E-51,1.,5.60383084497445E-34)) ;
#61629=DIRECTION('center_axis',(5.00382208281761E-15,1.,0.)) ;
#61630=DIRECTION('ref_axis',(1.,-5.00382208281761E-15,2.52374105052742E-18)) ;
#61631=DIRECTION('',(0.,0.,-1.)) ;
#61632=DIRECTION('center_axis',(1.,1.41426179436738E-51,0.)) ;
#61633=DIRECTION('ref_axis',(1.41426179436738E-51,-1.,-5.60383084497445E-34)) ;
#61634=DIRECTION('',(0.,0.,-1.)) ;
#61635=DIRECTION('center_axis',(0.,1.,0.)) ;
#61636=DIRECTION('ref_axis',(1.,0.,2.52374105052742E-18)) ;
#61637=DIRECTION('',(0.,0.,-1.)) ;
#61638=DIRECTION('center_axis',(-1.,7.65671051465623E-16,0.)) ;
#61639=DIRECTION('ref_axis',(7.65671051465623E-16,1.,2.49273854828173E-33)) ;
#61640=DIRECTION('',(0.,0.,-1.)) ;
#61641=DIRECTION('center_axis',(0.,-1.,0.)) ;
#61642=DIRECTION('ref_axis',(-1.,0.,-2.52374105052742E-18)) ;
#61643=DIRECTION('',(0.,0.,-1.)) ;
#61644=DIRECTION('center_axis',(-1.,-1.41426179436738E-51,0.)) ;
#61645=DIRECTION('ref_axis',(-1.41426179436738E-51,1.,5.60383084497445E-34)) ;
#86611=CARTESIAN_POINT('',(0.,0.,0.)) ;
#86612=CARTESIAN_POINT('Origin',(71.0296384056928,220.462610236549,30.6213203435596)) ;
#86613=CARTESIAN_POINT('',(66.535890167043,220.462610236549,30.7213203435596)) ;
#86614=CARTESIAN_POINT('',(66.5470607720161,220.362610236549,30.6213203435596)) ;
#86615=CARTESIAN_POINT('Ctrl Pts',(66.535890167043,220.462610236549,30.7213203435596)) ;
#86616=CARTESIAN_POINT('Ctrl Pts',(66.5375573265241,220.450073793375,30.7213203435596)) ;
#86617=CARTESIAN_POINT('Ctrl Pts',(66.5392266719142,220.436678341659,30.7188189533562)) ;
#86618=CARTESIAN_POINT('Ctrl Pts',(66.5421069063706,220.412004111391,30.7085970880789)) ;
#86619=CARTESIAN_POINT('Ctrl Pts',(66.5433203105337,220.400725238479,30.700877549635)) ;
#86620=CARTESIAN_POINT('Ctrl Pts',(66.5451460630584,220.382976586378,30.6830871681797)) ;
#86621=CARTESIAN_POINT('Ctrl Pts',(66.5458826827361,220.375300527803,30.6718610783706)) ;
#86622=CARTESIAN_POINT('Ctrl Pts',(66.5468387755779,220.365117510381,30.6472522185807)) ;
#86623=CARTESIAN_POINT('Ctrl Pts',(66.5470607720162,220.362610236549,30.633869677038)) ;
#86624=CARTESIAN_POINT('Ctrl Pts',(66.5470607720162,220.362610236549,30.6213203435596)) ;
#86625=CARTESIAN_POINT('',(72.0450953968557,220.362610236549,30.6213203435596)) ;
#86626=CARTESIAN_POINT('',(71.0296384056928,220.362610236549,30.6213203435596)) ;
#86627=CARTESIAN_POINT('',(72.0450953968557,220.462610236549,30.7213203435596)) ;
#86628=CARTESIAN_POINT('Origin',(72.0450953968557,220.462610236549,30.6213203435596)) ;
#86629=CARTESIAN_POINT('',(71.0296384056928,220.462610236549,30.7213203435596)) ;
#86630=CARTESIAN_POINT('Origin',(72.0450953968556,220.462610236549,30.7213203435596)) ;
#86631=CARTESIAN_POINT('',(72.1450953968557,220.462610236549,30.6213203435596)) ;
#86632=CARTESIAN_POINT('Origin',(72.0450953968556,220.462610236549,30.6213203435596)) ;
#86633=CARTESIAN_POINT('',(72.0450953968556,220.362610236549,29.6213203435596)) ;
#86634=CARTESIAN_POINT('',(72.0450953968556,220.362610236549,30.7213203435596)) ;
#86635=CARTESIAN_POINT('',(72.1450953968557,220.462610236549,29.6213203435596)) ;
#86636=CARTESIAN_POINT('Origin',(72.0450953968556,220.462610236549,29.6213203435596)) ;
#86637=CARTESIAN_POINT('',(72.1450953968557,220.462610236549,30.7213203435596)) ;
#86638=CARTESIAN_POINT('Origin',(71.0296384056928,220.462610236549,29.6213203435596)) ;
#86639=CARTESIAN_POINT('',(66.5470607720161,220.362610236549,29.6213203435596)) ;
#86640=CARTESIAN_POINT('',(66.535890167043,220.462610236549,29.5213203435596)) ;
#86641=CARTESIAN_POINT('Ctrl Pts',(66.5470607720162,220.362610236549,29.6213203435596)) ;
#86642=CARTESIAN_POINT('Ctrl Pts',(66.5470607720162,220.362610236549,29.6087513069564)) ;
#86643=CARTESIAN_POINT('Ctrl Pts',(66.5468380955723,220.365125326392,29.5953491152596)) ;
#86644=CARTESIAN_POINT('Ctrl Pts',(66.5458791440598,220.37533771967,29.5707102872029)) ;
#86645=CARTESIAN_POINT('Ctrl Pts',(66.5451403289395,220.383035341946,29.559473881925)) ;
#86646=CARTESIAN_POINT('Ctrl Pts',(66.5433118191149,220.400804731032,29.5417044928395)) ;
#86647=CARTESIAN_POINT('Ctrl Pts',(66.5420991240993,220.412073206815,29.5340065426202)) ;
#86648=CARTESIAN_POINT('Ctrl Pts',(66.5392218285232,220.436717456405,29.5238140042625)) ;
#86649=CARTESIAN_POINT('Ctrl Pts',(66.5375547295074,220.450093322012,29.5213203435596)) ;
#86650=CARTESIAN_POINT('Ctrl Pts',(66.535890167043,220.462610236549,29.5213203435596)) ;
#86651=CARTESIAN_POINT('',(72.0450953968557,220.462610236549,29.5213203435596)) ;
#86652=CARTESIAN_POINT('',(71.0296384056928,220.462610236549,29.5213203435596)) ;
#86653=CARTESIAN_POINT('Origin',(72.0450953968557,220.462610236549,29.6213203435596)) ;
#86654=CARTESIAN_POINT('',(71.0296384056928,220.362610236549,29.6213203435596)) ;
#86655=CARTESIAN_POINT('Origin',(72.0450953968557,220.462610236549,29.6213203435596)) ;
#86656=CARTESIAN_POINT('Origin',(72.0450953968557,220.462610236549,29.6213203435596)) ;
#86657=CARTESIAN_POINT('Origin',(72.0450953968557,220.462610236549,30.6213203435596)) ;
#86658=CARTESIAN_POINT('Origin',(72.0450953968557,220.462610236549,30.6213203435596)) ;
#86659=CARTESIAN_POINT('Origin',(69.9141814145298,238.377312217409,30.7213203435596)) ;
#86660=CARTESIAN_POINT('',(72.0450953968556,223.000000000001,30.7213203435596)) ;
#86661=CARTESIAN_POINT('',(72.0450953968556,230.688656108705,30.7213203435596)) ;
#86662=CARTESIAN_POINT('',(74.7,226.067880390059,30.7213203435596)) ;
#86663=CARTESIAN_POINT('Origin',(75.1450953968556,223.000000000001,30.7213203435596)) ;
#86664=CARTESIAN_POINT('',(74.7,231.000000000001,30.7213203435596)) ;
#86665=CARTESIAN_POINT('',(74.7,231.000000000001,30.7213203435596)) ;
#86666=CARTESIAN_POINT('',(79.0976680713511,231.000000000001,30.7213203435596)) ;
#86667=CARTESIAN_POINT('',(79.2,231.000000000001,30.7213203435596)) ;
#86668=CARTESIAN_POINT('',(80.1000000000001,235.614468918958,30.7213203435596)) ;
#86669=CARTESIAN_POINT('',(80.1582163984138,235.882481693345,30.7213203435596)) ;
#86670=CARTESIAN_POINT('',(80.1000000000001,238.703733341287,30.7213203435596)) ;
#86671=CARTESIAN_POINT('',(80.1000000000001,238.490522779348,30.7213203435596)) ;
#86672=CARTESIAN_POINT('',(82.1067384683691,238.703733341287,30.7213203435596)) ;
#86673=CARTESIAN_POINT('',(76.057090707265,238.703733341287,30.7213203435596)) ;
#86674=CARTESIAN_POINT('',(82.183342912681,238.739454580319,30.7213203435596)) ;
#86675=CARTESIAN_POINT('Origin',(82.1067384683691,238.803733341287,30.7213203435596)) ;
#86676=CARTESIAN_POINT('',(83.9347806063073,240.826736743903,30.7213203435596)) ;
#86677=CARTESIAN_POINT('',(80.4937295064186,236.72585173331,30.7213203435596)) ;
#86678=CARTESIAN_POINT('',(84.0283628290597,241.083851787777,30.7213203435596)) ;
#86679=CARTESIAN_POINT('Origin',(83.6283628290597,241.083851787777,30.7213203435596)) ;
#86680=CARTESIAN_POINT('',(84.0283628290597,244.119881553511,30.7213203435596)) ;
#86681=CARTESIAN_POINT('',(84.0283628290597,241.339589444027,30.7213203435596)) ;
#86682=CARTESIAN_POINT('',(83.9347806063073,244.376996597386,30.7213203435596)) ;
#86683=CARTESIAN_POINT('Origin',(83.6283628290597,244.119881553511,30.7213203435596)) ;
#86684=CARTESIAN_POINT('',(82.2732639481701,246.357115043876,30.7213203435596)) ;
#86685=CARTESIAN_POINT('',(81.6097350811727,247.14787795491,30.7213203435596)) ;
#86686=CARTESIAN_POINT('',(81.9668461709225,246.500000000001,30.7213203435596)) ;
#86687=CARTESIAN_POINT('Origin',(81.9668461709225,246.100000000001,30.7213203435596)) ;
#86688=CARTESIAN_POINT('',(79.1,246.500000000001,30.7213203435596)) ;
#86689=CARTESIAN_POINT('',(74.5570907072649,246.500000000001,30.7213203435596)) ;
#86690=CARTESIAN_POINT('',(79.1,253.900000000001,30.7213203435596)) ;
#86691=CARTESIAN_POINT('',(79.1,246.138656108705,30.7213203435596)) ;
#86692=CARTESIAN_POINT('',(67.6,253.900000000001,30.7213203435596)) ;
#86693=CARTESIAN_POINT('',(67.6,253.900000000001,30.7213203435596)) ;
#86694=CARTESIAN_POINT('',(67.6,257.5,30.7213203435596)) ;
#86695=CARTESIAN_POINT('',(67.6,257.5,30.7213203435596)) ;
#86696=CARTESIAN_POINT('',(55.7,257.5,30.7213203435596)) ;
#86697=CARTESIAN_POINT('',(55.7,257.5,30.7213203435596)) ;
#86698=CARTESIAN_POINT('',(55.7,245.9,30.7213203435596)) ;
#86699=CARTESIAN_POINT('',(55.7,245.9,30.7213203435596)) ;
#86700=CARTESIAN_POINT('',(58.9573593128807,245.9,30.7213203435596)) ;
#86701=CARTESIAN_POINT('',(58.9573593128807,245.9,30.7213203435596)) ;
#86702=CARTESIAN_POINT('',(58.9573593128807,226.1,30.7213203435596)) ;
#86703=CARTESIAN_POINT('',(58.9573593128807,239.1,30.7213203435596)) ;
#86704=CARTESIAN_POINT('',(61.775147916658,220.442149698512,30.7213203435596)) ;
#86705=CARTESIAN_POINT('',(58.9573593128807,226.1,30.7213203435596)) ;
#86706=CARTESIAN_POINT('Origin',(64.1568347953872,220.146231446812,30.7213203435596)) ;
#86707=CARTESIAN_POINT('',(75.3756995384723,242.900000000001,30.7213203435596)) ;
#86708=CARTESIAN_POINT('',(75.3756995384723,240.900000000001,30.7213203435596)) ;
#86709=CARTESIAN_POINT('',(75.3756995384723,240.638656108705,30.7213203435596)) ;
#86710=CARTESIAN_POINT('',(78.481026119647,242.900000000001,30.7213203435596)) ;
#86711=CARTESIAN_POINT('Origin',(76.9283628290597,242.900000000001,30.7213203435596)) ;
#86712=CARTESIAN_POINT('',(78.481026119647,240.900000000001,30.7213203435596)) ;
#86713=CARTESIAN_POINT('',(78.481026119647,239.638656108705,30.7213203435596)) ;
#86714=CARTESIAN_POINT('Origin',(76.9283628290597,240.900000000001,30.7213203435596)) ;
#86715=CARTESIAN_POINT('',(73.9,229.6,30.7213203435596)) ;
#86716=CARTESIAN_POINT('',(74.2,229.90139888331,30.7213203435596)) ;
#86717=CARTESIAN_POINT('Ctrl Pts',(74.2,229.90139888331,30.7213203435596)) ;
#86718=CARTESIAN_POINT('Ctrl Pts',(74.2,229.864103877398,30.7213203435596)) ;
#86719=CARTESIAN_POINT('Ctrl Pts',(74.1913108545003,229.820201486786,30.7213203435596)) ;
#86720=CARTESIAN_POINT('Ctrl Pts',(74.1628856418395,229.751400609842,30.7213203435596)) ;
#86721=CARTESIAN_POINT('Ctrl Pts',(74.1381754797833,229.714300461156,30.7213203435596)) ;
#86722=CARTESIAN_POINT('Ctrl Pts',(74.0857759852183,229.661783948368,30.7213203435596)) ;
#86723=CARTESIAN_POINT('Ctrl Pts',(74.0488482525377,229.637045411928,30.7213203435596)) ;
#86724=CARTESIAN_POINT('Ctrl Pts',(73.9804869087102,229.608675189374,30.7213203435596)) ;
#86725=CARTESIAN_POINT('Ctrl Pts',(73.9369742156035,229.6,30.7213203435596)) ;
#86726=CARTESIAN_POINT('Ctrl Pts',(73.9,229.6,30.7213203435596)) ;
#86727=CARTESIAN_POINT('',(72.1,229.6,30.7213203435596)) ;
#86728=CARTESIAN_POINT('',(74.2,229.6,30.7213203435596)) ;
#86729=CARTESIAN_POINT('',(71.8,229.90139888331,30.7213203435596)) ;
#86730=CARTESIAN_POINT('Ctrl Pts',(72.1,229.6,30.7213203435596)) ;
#86731=CARTESIAN_POINT('Ctrl Pts',(72.0630257843965,229.6,30.7213203435596)) ;
#86732=CARTESIAN_POINT('Ctrl Pts',(72.0195130912898,229.608675189374,30.7213203435596)) ;
#86733=CARTESIAN_POINT('Ctrl Pts',(71.9511517474623,229.637045411928,30.7213203435596)) ;
#86734=CARTESIAN_POINT('Ctrl Pts',(71.9142240147817,229.661783948368,30.7213203435596)) ;
#86735=CARTESIAN_POINT('Ctrl Pts',(71.8618245202167,229.714300461156,30.7213203435596)) ;
#86736=CARTESIAN_POINT('Ctrl Pts',(71.8371143581605,229.751400609842,30.7213203435596)) ;
#86737=CARTESIAN_POINT('Ctrl Pts',(71.8086891454997,229.820201486786,30.7213203435596)) ;
#86738=CARTESIAN_POINT('Ctrl Pts',(71.8,229.864103877398,30.7213203435596)) ;
#86739=CARTESIAN_POINT('Ctrl Pts',(71.8,229.90139888331,30.7213203435596)) ;
#86740=CARTESIAN_POINT('',(71.8,231.69860111669,30.7213203435596)) ;
#86741=CARTESIAN_POINT('',(71.8,229.6,30.7213203435596)) ;
#86742=CARTESIAN_POINT('',(72.1,232.,30.7213203435596)) ;
#86743=CARTESIAN_POINT('Ctrl Pts',(71.8,231.69860111669,30.7213203435596)) ;
#86744=CARTESIAN_POINT('Ctrl Pts',(71.8,231.735896122602,30.7213203435596)) ;
#86745=CARTESIAN_POINT('Ctrl Pts',(71.8086891454997,231.779798513214,30.7213203435596)) ;
#86746=CARTESIAN_POINT('Ctrl Pts',(71.8371143581605,231.848599390158,30.7213203435596)) ;
#86747=CARTESIAN_POINT('Ctrl Pts',(71.8618245202167,231.885699538844,30.7213203435596)) ;
#86748=CARTESIAN_POINT('Ctrl Pts',(71.9142240147817,231.938216051632,30.7213203435596)) ;
#86749=CARTESIAN_POINT('Ctrl Pts',(71.9511517474623,231.962954588072,30.7213203435596)) ;
#86750=CARTESIAN_POINT('Ctrl Pts',(72.0195130912898,231.991324810626,30.7213203435596)) ;
#86751=CARTESIAN_POINT('Ctrl Pts',(72.0630257843965,232.,30.7213203435596)) ;
#86752=CARTESIAN_POINT('Ctrl Pts',(72.1,232.,30.7213203435596)) ;
#86753=CARTESIAN_POINT('',(73.9,232.,30.7213203435596)) ;
#86754=CARTESIAN_POINT('',(71.8,232.,30.7213203435596)) ;
#86755=CARTESIAN_POINT('',(74.2,231.69860111669,30.7213203435596)) ;
#86756=CARTESIAN_POINT('Ctrl Pts',(73.9,232.,30.7213203435596)) ;
#86757=CARTESIAN_POINT('Ctrl Pts',(73.9369742156035,232.,30.7213203435596)) ;
#86758=CARTESIAN_POINT('Ctrl Pts',(73.9804869087102,231.991324810626,30.7213203435596)) ;
#86759=CARTESIAN_POINT('Ctrl Pts',(74.0488482525377,231.962954588072,30.7213203435596)) ;
#86760=CARTESIAN_POINT('Ctrl Pts',(74.0857759852183,231.938216051632,30.7213203435596)) ;
#86761=CARTESIAN_POINT('Ctrl Pts',(74.1381754797833,231.885699538844,30.7213203435596)) ;
#86762=CARTESIAN_POINT('Ctrl Pts',(74.1628856418395,231.848599390158,30.7213203435596)) ;
#86763=CARTESIAN_POINT('Ctrl Pts',(74.1913108545003,231.779798513214,30.7213203435596)) ;
#86764=CARTESIAN_POINT('Ctrl Pts',(74.2,231.735896122602,30.7213203435596)) ;
#86765=CARTESIAN_POINT('Ctrl Pts',(74.2,231.69860111669,30.7213203435596)) ;
#86766=CARTESIAN_POINT('',(74.2,232.,30.7213203435596)) ;
#86767=CARTESIAN_POINT('',(66.8,254.6,30.7213203435596)) ;
#86768=CARTESIAN_POINT('',(65.,254.6,30.7213203435596)) ;
#86769=CARTESIAN_POINT('',(67.3070907072649,254.6,30.7213203435596)) ;
#86770=CARTESIAN_POINT('',(64.7,254.90139888331,30.7213203435596)) ;
#86771=CARTESIAN_POINT('Ctrl Pts',(65.,254.6,30.7213203435596)) ;
#86772=CARTESIAN_POINT('Ctrl Pts',(64.9630257843965,254.6,30.7213203435596)) ;
#86773=CARTESIAN_POINT('Ctrl Pts',(64.9195130912898,254.608675189374,30.7213203435596)) ;
#86774=CARTESIAN_POINT('Ctrl Pts',(64.8511517474623,254.637045411928,30.7213203435596)) ;
#86775=CARTESIAN_POINT('Ctrl Pts',(64.8142240147817,254.661783948368,30.7213203435596)) ;
#86776=CARTESIAN_POINT('Ctrl Pts',(64.7618245202167,254.714300461156,30.7213203435596)) ;
#86777=CARTESIAN_POINT('Ctrl Pts',(64.7371143581605,254.751400609842,30.7213203435596)) ;
#86778=CARTESIAN_POINT('Ctrl Pts',(64.7086891454997,254.820201486786,30.7213203435596)) ;
#86779=CARTESIAN_POINT('Ctrl Pts',(64.7,254.864103877398,30.7213203435596)) ;
#86780=CARTESIAN_POINT('Ctrl Pts',(64.7,254.90139888331,30.7213203435596)) ;
#86781=CARTESIAN_POINT('',(64.7,256.69860111669,30.7213203435596)) ;
#86782=CARTESIAN_POINT('',(64.7,247.688656108704,30.7213203435596)) ;
#86783=CARTESIAN_POINT('',(65.,257.,30.7213203435596)) ;
#86784=CARTESIAN_POINT('Ctrl Pts',(64.7,256.69860111669,30.7213203435596)) ;
#86785=CARTESIAN_POINT('Ctrl Pts',(64.7,256.735896122602,30.7213203435596)) ;
#86786=CARTESIAN_POINT('Ctrl Pts',(64.7086891454997,256.779798513214,30.7213203435596)) ;
#86787=CARTESIAN_POINT('Ctrl Pts',(64.7371143581605,256.848599390158,30.7213203435596)) ;
#86788=CARTESIAN_POINT('Ctrl Pts',(64.7618245202167,256.885699538844,30.7213203435596)) ;
#86789=CARTESIAN_POINT('Ctrl Pts',(64.8142240147817,256.938216051632,30.7213203435596)) ;
#86790=CARTESIAN_POINT('Ctrl Pts',(64.8511517474623,256.962954588072,30.7213203435596)) ;
#86791=CARTESIAN_POINT('Ctrl Pts',(64.9195130912898,256.991324810626,30.7213203435596)) ;
#86792=CARTESIAN_POINT('Ctrl Pts',(64.9630257843965,257.,30.7213203435596)) ;
#86793=CARTESIAN_POINT('Ctrl Pts',(65.,257.,30.7213203435596)) ;
#86794=CARTESIAN_POINT('',(66.8,257.,30.7213203435596)) ;
#86795=CARTESIAN_POINT('',(68.5070907072649,257.,30.7213203435596)) ;
#86796=CARTESIAN_POINT('',(67.1,256.69860111669,30.7213203435596)) ;
#86797=CARTESIAN_POINT('Ctrl Pts',(66.8,257.,30.7213203435596)) ;
#86798=CARTESIAN_POINT('Ctrl Pts',(66.8369742156035,257.,30.7213203435596)) ;
#86799=CARTESIAN_POINT('Ctrl Pts',(66.8804869087102,256.991324810626,30.7213203435596)) ;
#86800=CARTESIAN_POINT('Ctrl Pts',(66.9488482525377,256.962954588072,30.7213203435596)) ;
#86801=CARTESIAN_POINT('Ctrl Pts',(66.9857759852183,256.938216051632,30.7213203435596)) ;
#86802=CARTESIAN_POINT('Ctrl Pts',(67.0381754797833,256.885699538844,30.7213203435596)) ;
#86803=CARTESIAN_POINT('Ctrl Pts',(67.0628856418395,256.848599390158,30.7213203435596)) ;
#86804=CARTESIAN_POINT('Ctrl Pts',(67.0913108545003,256.779798513214,30.7213203435596)) ;
#86805=CARTESIAN_POINT('Ctrl Pts',(67.1,256.735896122602,30.7213203435596)) ;
#86806=CARTESIAN_POINT('Ctrl Pts',(67.1,256.69860111669,30.7213203435596)) ;
#86807=CARTESIAN_POINT('',(67.1,254.90139888331,30.7213203435596)) ;
#86808=CARTESIAN_POINT('',(67.1,246.488656108704,30.7213203435596)) ;
#86809=CARTESIAN_POINT('Ctrl Pts',(67.1,254.90139888331,30.7213203435596)) ;
#86810=CARTESIAN_POINT('Ctrl Pts',(67.1,254.864103877398,30.7213203435596)) ;
#86811=CARTESIAN_POINT('Ctrl Pts',(67.0913108545003,254.820201486786,30.7213203435596)) ;
#86812=CARTESIAN_POINT('Ctrl Pts',(67.0628856418395,254.751400609842,30.7213203435596)) ;
#86813=CARTESIAN_POINT('Ctrl Pts',(67.0381754797833,254.714300461156,30.7213203435596)) ;
#86814=CARTESIAN_POINT('Ctrl Pts',(66.9857759852183,254.661783948368,30.7213203435596)) ;
#86815=CARTESIAN_POINT('Ctrl Pts',(66.9488482525377,254.637045411928,30.7213203435596)) ;
#86816=CARTESIAN_POINT('Ctrl Pts',(66.8804869087102,254.608675189374,30.7213203435596)) ;
#86817=CARTESIAN_POINT('Ctrl Pts',(66.8369742156035,254.6,30.7213203435596)) ;
#86818=CARTESIAN_POINT('Ctrl Pts',(66.8,254.6,30.7213203435596)) ;
#86819=CARTESIAN_POINT('',(62.0573593128807,233.6,30.7213203435596)) ;
#86820=CARTESIAN_POINT('',(60.2573593128808,233.6,30.7213203435596)) ;
#86821=CARTESIAN_POINT('',(64.9357703637053,233.6,30.7213203435596)) ;
#86822=CARTESIAN_POINT('',(59.9573593128807,233.90139888331,30.7213203435596)) ;
#86823=CARTESIAN_POINT('Ctrl Pts',(60.2573593128808,233.6,30.7213203435596)) ;
#86824=CARTESIAN_POINT('Ctrl Pts',(60.2203850972773,233.6,30.7213203435596)) ;
#86825=CARTESIAN_POINT('Ctrl Pts',(60.1768724041706,233.608675189374,30.7213203435596)) ;
#86826=CARTESIAN_POINT('Ctrl Pts',(60.1085110603431,233.637045411928,30.7213203435596)) ;
#86827=CARTESIAN_POINT('Ctrl Pts',(60.0715833276625,233.661783948368,30.7213203435596)) ;
#86828=CARTESIAN_POINT('Ctrl Pts',(60.0191838330975,233.714300461156,30.7213203435596)) ;
#86829=CARTESIAN_POINT('Ctrl Pts',(59.9944736710413,233.751400609842,30.7213203435596)) ;
#86830=CARTESIAN_POINT('Ctrl Pts',(59.9660484583805,233.820201486786,30.7213203435596)) ;
#86831=CARTESIAN_POINT('Ctrl Pts',(59.9573593128808,233.864103877398,30.7213203435596)) ;
#86832=CARTESIAN_POINT('Ctrl Pts',(59.9573593128808,233.90139888331,30.7213203435596)) ;
#86833=CARTESIAN_POINT('',(59.9573593128807,235.69860111669,30.7213203435596)) ;
#86834=CARTESIAN_POINT('',(59.9573593128807,237.188656108704,30.7213203435596)) ;
#86835=CARTESIAN_POINT('',(60.2573593128808,236.,30.7213203435596)) ;
#86836=CARTESIAN_POINT('Ctrl Pts',(59.9573593128808,235.69860111669,30.7213203435596)) ;
#86837=CARTESIAN_POINT('Ctrl Pts',(59.9573593128808,235.735896122602,30.7213203435596)) ;
#86838=CARTESIAN_POINT('Ctrl Pts',(59.9660484583805,235.779798513214,30.7213203435596)) ;
#86839=CARTESIAN_POINT('Ctrl Pts',(59.9944736710413,235.848599390158,30.7213203435596)) ;
#86840=CARTESIAN_POINT('Ctrl Pts',(60.0191838330975,235.885699538844,30.7213203435596)) ;
#86841=CARTESIAN_POINT('Ctrl Pts',(60.0715833276625,235.938216051632,30.7213203435596)) ;
#86842=CARTESIAN_POINT('Ctrl Pts',(60.1085110603431,235.962954588072,30.7213203435596)) ;
#86843=CARTESIAN_POINT('Ctrl Pts',(60.1768724041706,235.991324810626,30.7213203435596)) ;
#86844=CARTESIAN_POINT('Ctrl Pts',(60.2203850972773,236.,30.7213203435596)) ;
#86845=CARTESIAN_POINT('Ctrl Pts',(60.2573593128808,236.,30.7213203435596)) ;
#86846=CARTESIAN_POINT('',(62.0573593128807,236.,30.7213203435596)) ;
#86847=CARTESIAN_POINT('',(66.1357703637053,236.,30.7213203435596)) ;
#86848=CARTESIAN_POINT('',(62.3573593128808,235.69860111669,30.7213203435596)) ;
#86849=CARTESIAN_POINT('Ctrl Pts',(62.0573593128807,236.,30.7213203435596)) ;
#86850=CARTESIAN_POINT('Ctrl Pts',(62.0943335284842,236.,30.7213203435596)) ;
#86851=CARTESIAN_POINT('Ctrl Pts',(62.1378462215909,235.991324810626,30.7213203435596)) ;
#86852=CARTESIAN_POINT('Ctrl Pts',(62.2062075654184,235.962954588072,30.7213203435596)) ;
#86853=CARTESIAN_POINT('Ctrl Pts',(62.243135298099,235.938216051632,30.7213203435596)) ;
#86854=CARTESIAN_POINT('Ctrl Pts',(62.295534792664,235.885699538844,30.7213203435596)) ;
#86855=CARTESIAN_POINT('Ctrl Pts',(62.3202449547202,235.848599390158,30.7213203435596)) ;
#86856=CARTESIAN_POINT('Ctrl Pts',(62.348670167381,235.779798513214,30.7213203435596)) ;
#86857=CARTESIAN_POINT('Ctrl Pts',(62.3573593128807,235.735896122602,30.7213203435596)) ;
#86858=CARTESIAN_POINT('Ctrl Pts',(62.3573593128807,235.69860111669,30.7213203435596)) ;
#86859=CARTESIAN_POINT('',(62.3573593128808,233.90139888331,30.7213203435596)) ;
#86860=CARTESIAN_POINT('',(62.3573593128808,235.988656108704,30.7213203435596)) ;
#86861=CARTESIAN_POINT('Ctrl Pts',(62.3573593128807,233.90139888331,30.7213203435596)) ;
#86862=CARTESIAN_POINT('Ctrl Pts',(62.3573593128807,233.864103877398,30.7213203435596)) ;
#86863=CARTESIAN_POINT('Ctrl Pts',(62.348670167381,233.820201486786,30.7213203435596)) ;
#86864=CARTESIAN_POINT('Ctrl Pts',(62.3202449547202,233.751400609842,30.7213203435596)) ;
#86865=CARTESIAN_POINT('Ctrl Pts',(62.295534792664,233.714300461156,30.7213203435596)) ;
#86866=CARTESIAN_POINT('Ctrl Pts',(62.243135298099,233.661783948368,30.7213203435596)) ;
#86867=CARTESIAN_POINT('Ctrl Pts',(62.2062075654184,233.637045411928,30.7213203435596)) ;
#86868=CARTESIAN_POINT('Ctrl Pts',(62.1378462215909,233.608675189374,30.7213203435596)) ;
#86869=CARTESIAN_POINT('Ctrl Pts',(62.0943335284842,233.6,30.7213203435596)) ;
#86870=CARTESIAN_POINT('Ctrl Pts',(62.0573593128807,233.6,30.7213203435596)) ;
#86871=CARTESIAN_POINT('',(58.8,254.6,30.7213203435596)) ;
#86872=CARTESIAN_POINT('',(57.,254.6,30.7213203435596)) ;
#86873=CARTESIAN_POINT('',(63.3070907072649,254.6,30.7213203435596)) ;
#86874=CARTESIAN_POINT('',(56.7,254.90139888331,30.7213203435596)) ;
#86875=CARTESIAN_POINT('Ctrl Pts',(57.,254.6,30.7213203435596)) ;
#86876=CARTESIAN_POINT('Ctrl Pts',(56.9630257843965,254.6,30.7213203435596)) ;
#86877=CARTESIAN_POINT('Ctrl Pts',(56.9195130912898,254.608675189374,30.7213203435596)) ;
#86878=CARTESIAN_POINT('Ctrl Pts',(56.8511517474623,254.637045411928,30.7213203435596)) ;
#86879=CARTESIAN_POINT('Ctrl Pts',(56.8142240147817,254.661783948368,30.7213203435596)) ;
#86880=CARTESIAN_POINT('Ctrl Pts',(56.7618245202167,254.714300461156,30.7213203435596)) ;
#86881=CARTESIAN_POINT('Ctrl Pts',(56.7371143581605,254.751400609842,30.7213203435596)) ;
#86882=CARTESIAN_POINT('Ctrl Pts',(56.7086891454997,254.820201486786,30.7213203435596)) ;
#86883=CARTESIAN_POINT('Ctrl Pts',(56.7,254.864103877398,30.7213203435596)) ;
#86884=CARTESIAN_POINT('Ctrl Pts',(56.7,254.90139888331,30.7213203435596)) ;
#86885=CARTESIAN_POINT('',(56.7,256.69860111669,30.7213203435596)) ;
#86886=CARTESIAN_POINT('',(56.7,247.688656108704,30.7213203435596)) ;
#86887=CARTESIAN_POINT('',(57.,257.,30.7213203435596)) ;
#86888=CARTESIAN_POINT('Ctrl Pts',(56.7,256.69860111669,30.7213203435596)) ;
#86889=CARTESIAN_POINT('Ctrl Pts',(56.7,256.735896122602,30.7213203435596)) ;
#86890=CARTESIAN_POINT('Ctrl Pts',(56.7086891454997,256.779798513214,30.7213203435596)) ;
#86891=CARTESIAN_POINT('Ctrl Pts',(56.7371143581605,256.848599390158,30.7213203435596)) ;
#86892=CARTESIAN_POINT('Ctrl Pts',(56.7618245202167,256.885699538844,30.7213203435596)) ;
#86893=CARTESIAN_POINT('Ctrl Pts',(56.8142240147817,256.938216051632,30.7213203435596)) ;
#86894=CARTESIAN_POINT('Ctrl Pts',(56.8511517474623,256.962954588072,30.7213203435596)) ;
#86895=CARTESIAN_POINT('Ctrl Pts',(56.9195130912898,256.991324810626,30.7213203435596)) ;
#86896=CARTESIAN_POINT('Ctrl Pts',(56.9630257843965,257.,30.7213203435596)) ;
#86897=CARTESIAN_POINT('Ctrl Pts',(57.,257.,30.7213203435596)) ;
#86898=CARTESIAN_POINT('',(58.8,257.,30.7213203435596)) ;
#86899=CARTESIAN_POINT('',(64.5070907072649,257.,30.7213203435596)) ;
#86900=CARTESIAN_POINT('',(59.1,256.69860111669,30.7213203435596)) ;
#86901=CARTESIAN_POINT('Ctrl Pts',(58.8,257.,30.7213203435596)) ;
#86902=CARTESIAN_POINT('Ctrl Pts',(58.8369742156035,257.,30.7213203435596)) ;
#86903=CARTESIAN_POINT('Ctrl Pts',(58.8804869087102,256.991324810626,30.7213203435596)) ;
#86904=CARTESIAN_POINT('Ctrl Pts',(58.9488482525377,256.962954588072,30.7213203435596)) ;
#86905=CARTESIAN_POINT('Ctrl Pts',(58.9857759852183,256.938216051632,30.7213203435596)) ;
#86906=CARTESIAN_POINT('Ctrl Pts',(59.0381754797833,256.885699538844,30.7213203435596)) ;
#86907=CARTESIAN_POINT('Ctrl Pts',(59.0628856418395,256.848599390158,30.7213203435596)) ;
#86908=CARTESIAN_POINT('Ctrl Pts',(59.0913108545003,256.779798513214,30.7213203435596)) ;
#86909=CARTESIAN_POINT('Ctrl Pts',(59.1,256.735896122602,30.7213203435596)) ;
#86910=CARTESIAN_POINT('Ctrl Pts',(59.1,256.69860111669,30.7213203435596)) ;
#86911=CARTESIAN_POINT('',(59.1,254.90139888331,30.7213203435596)) ;
#86912=CARTESIAN_POINT('',(59.1,246.488656108705,30.7213203435596)) ;
#86913=CARTESIAN_POINT('Ctrl Pts',(59.1,254.90139888331,30.7213203435596)) ;
#86914=CARTESIAN_POINT('Ctrl Pts',(59.1,254.864103877398,30.7213203435596)) ;
#86915=CARTESIAN_POINT('Ctrl Pts',(59.0913108545003,254.820201486786,30.7213203435596)) ;
#86916=CARTESIAN_POINT('Ctrl Pts',(59.0628856418395,254.751400609842,30.7213203435596)) ;
#86917=CARTESIAN_POINT('Ctrl Pts',(59.0381754797833,254.714300461156,30.7213203435596)) ;
#86918=CARTESIAN_POINT('Ctrl Pts',(58.9857759852183,254.661783948368,30.7213203435596)) ;
#86919=CARTESIAN_POINT('Ctrl Pts',(58.9488482525377,254.637045411928,30.7213203435596)) ;
#86920=CARTESIAN_POINT('Ctrl Pts',(58.8804869087102,254.608675189374,30.7213203435596)) ;
#86921=CARTESIAN_POINT('Ctrl Pts',(58.8369742156035,254.6,30.7213203435596)) ;
#86922=CARTESIAN_POINT('Ctrl Pts',(58.8,254.6,30.7213203435596)) ;
#86923=CARTESIAN_POINT('Origin',(72.0450953968556,230.688656108705,30.6213203435596)) ;
#86924=CARTESIAN_POINT('',(72.1450953968556,223.000000000001,30.6213203435596)) ;
#86925=CARTESIAN_POINT('',(72.1450953968556,230.688656108705,30.6213203435596)) ;
#86926=CARTESIAN_POINT('Origin',(72.0450953968556,223.000000000001,30.6213203435596)) ;
#86927=CARTESIAN_POINT('Origin',(72.1450953968556,223.000000000001,30.7213203435596)) ;
#86928=CARTESIAN_POINT('',(72.1450953968556,223.000000000001,29.6213203435596)) ;
#86929=CARTESIAN_POINT('',(72.1450953968556,230.688656108705,29.6213203435596)) ;
#86930=CARTESIAN_POINT('',(72.1450953968556,223.000000000001,30.7213203435596)) ;
#86931=CARTESIAN_POINT('Origin',(72.0450953968556,230.688656108705,29.6213203435596)) ;
#86932=CARTESIAN_POINT('',(72.0450953968556,223.000000000001,29.5213203435596)) ;
#86933=CARTESIAN_POINT('',(72.0450953968556,230.688656108705,29.5213203435596)) ;
#86934=CARTESIAN_POINT('Origin',(72.0450953968556,223.000000000001,29.6213203435596)) ;
#86935=CARTESIAN_POINT('Origin',(69.9141814145298,238.377312217409,29.5213203435596)) ;
#86936=CARTESIAN_POINT('',(61.775147916658,220.442149698512,29.5213203435596)) ;
#86937=CARTESIAN_POINT('Origin',(64.1568347953872,220.146231446812,29.5213203435596)) ;
#86938=CARTESIAN_POINT('',(58.9573593128807,226.1,29.5213203435596)) ;
#86939=CARTESIAN_POINT('',(58.9573593128807,226.1,29.5213203435596)) ;
#86940=CARTESIAN_POINT('',(58.9573593128807,245.9,29.5213203435596)) ;
#86941=CARTESIAN_POINT('',(58.9573593128807,239.1,29.5213203435596)) ;
#86942=CARTESIAN_POINT('',(55.7,245.9,29.5213203435596)) ;
#86943=CARTESIAN_POINT('',(58.9573593128807,245.9,29.5213203435596)) ;
#86944=CARTESIAN_POINT('',(55.7,257.5,29.5213203435596)) ;
#86945=CARTESIAN_POINT('',(55.7,245.9,29.5213203435596)) ;
#86946=CARTESIAN_POINT('',(67.6,257.5,29.5213203435596)) ;
#86947=CARTESIAN_POINT('',(55.7,257.5,29.5213203435596)) ;
#86948=CARTESIAN_POINT('',(67.6,253.900000000001,29.5213203435596)) ;
#86949=CARTESIAN_POINT('',(67.6,257.5,29.5213203435596)) ;
#86950=CARTESIAN_POINT('',(79.1,253.900000000001,29.5213203435596)) ;
#86951=CARTESIAN_POINT('',(67.6,253.900000000001,29.5213203435596)) ;
#86952=CARTESIAN_POINT('',(79.1,246.500000000001,29.5213203435596)) ;
#86953=CARTESIAN_POINT('',(79.1,246.138656108705,29.5213203435596)) ;
#86954=CARTESIAN_POINT('',(81.9668461709225,246.500000000001,29.5213203435596)) ;
#86955=CARTESIAN_POINT('',(74.5570907072649,246.500000000001,29.5213203435596)) ;
#86956=CARTESIAN_POINT('',(82.2732639481701,246.357115043876,29.5213203435596)) ;
#86957=CARTESIAN_POINT('Origin',(81.9668461709225,246.100000000001,29.5213203435596)) ;
#86958=CARTESIAN_POINT('',(83.9347806063073,244.376996597386,29.5213203435596)) ;
#86959=CARTESIAN_POINT('',(81.6097350811727,247.14787795491,29.5213203435596)) ;
#86960=CARTESIAN_POINT('',(84.0283628290597,244.119881553511,29.5213203435596)) ;
#86961=CARTESIAN_POINT('Origin',(83.6283628290597,244.119881553511,29.5213203435596)) ;
#86962=CARTESIAN_POINT('',(84.0283628290597,241.083851787777,29.5213203435596)) ;
#86963=CARTESIAN_POINT('',(84.0283628290597,241.339589444027,29.5213203435596)) ;
#86964=CARTESIAN_POINT('',(83.9347806063073,240.826736743903,29.5213203435596)) ;
#86965=CARTESIAN_POINT('Origin',(83.6283628290597,241.083851787777,29.5213203435596)) ;
#86966=CARTESIAN_POINT('',(82.183342912681,238.739454580319,29.5213203435596)) ;
#86967=CARTESIAN_POINT('',(80.4937295064186,236.72585173331,29.5213203435596)) ;
#86968=CARTESIAN_POINT('',(82.1067384683691,238.703733341287,29.5213203435596)) ;
#86969=CARTESIAN_POINT('Origin',(82.1067384683691,238.803733341287,29.5213203435596)) ;
#86970=CARTESIAN_POINT('',(80.1000000000001,238.703733341287,29.5213203435596)) ;
#86971=CARTESIAN_POINT('',(76.057090707265,238.703733341287,29.5213203435596)) ;
#86972=CARTESIAN_POINT('',(80.1000000000001,235.614468918958,29.5213203435596)) ;
#86973=CARTESIAN_POINT('',(80.1000000000001,238.490522779348,29.5213203435596)) ;
#86974=CARTESIAN_POINT('',(79.0976680713511,231.000000000001,29.5213203435596)) ;
#86975=CARTESIAN_POINT('',(80.1582163984138,235.882481693345,29.5213203435596)) ;
#86976=CARTESIAN_POINT('',(74.7,231.000000000001,29.5213203435596)) ;
#86977=CARTESIAN_POINT('',(79.2,231.000000000001,29.5213203435596)) ;
#86978=CARTESIAN_POINT('',(74.7,226.067880390059,29.5213203435596)) ;
#86979=CARTESIAN_POINT('',(74.7,231.000000000001,29.5213203435596)) ;
#86980=CARTESIAN_POINT('Origin',(75.1450953968556,223.000000000001,29.5213203435596)) ;
#86981=CARTESIAN_POINT('',(78.381026119647,242.900000000001,29.5213203435596)) ;
#86982=CARTESIAN_POINT('',(75.4756995384723,242.900000000001,29.5213203435596)) ;
#86983=CARTESIAN_POINT('Origin',(76.9283628290597,242.900000000001,29.5213203435596)) ;
#86984=CARTESIAN_POINT('',(75.4756995384723,240.900000000001,29.5213203435596)) ;
#86985=CARTESIAN_POINT('',(75.4756995384723,240.900000000001,29.5213203435596)) ;
#86986=CARTESIAN_POINT('',(78.381026119647,240.900000000001,29.5213203435596)) ;
#86987=CARTESIAN_POINT('Origin',(76.9283628290597,240.900000000001,29.5213203435596)) ;
#86988=CARTESIAN_POINT('',(78.381026119647,242.900000000001,29.5213203435596)) ;
#86989=CARTESIAN_POINT('',(74.2,229.6,29.5213203435596)) ;
#86990=CARTESIAN_POINT('',(74.2,232.,29.5213203435596)) ;
#86991=CARTESIAN_POINT('',(74.2,232.,29.5213203435596)) ;
#86992=CARTESIAN_POINT('',(71.8,232.,29.5213203435596)) ;
#86993=CARTESIAN_POINT('',(71.8,232.,29.5213203435596)) ;
#86994=CARTESIAN_POINT('',(71.8,229.6,29.5213203435596)) ;
#86995=CARTESIAN_POINT('',(71.8,229.6,29.5213203435596)) ;
#86996=CARTESIAN_POINT('',(74.2,229.6,29.5213203435596)) ;
#86997=CARTESIAN_POINT('Origin',(79.1,246.138656108705,29.6213203435596)) ;
#86998=CARTESIAN_POINT('',(79.2,253.900000000001,29.6213203435596)) ;
#86999=CARTESIAN_POINT('Origin',(79.1,253.900000000001,29.6213203435596)) ;
#87000=CARTESIAN_POINT('',(79.2,246.600000000001,29.6213203435596)) ;
#87001=CARTESIAN_POINT('',(79.2,246.138656108705,29.6213203435596)) ;
#87002=CARTESIAN_POINT('Origin',(79.1,246.500000000001,29.6213203435596)) ;
#87003=CARTESIAN_POINT('Origin',(79.1,246.138656108705,30.6213203435596)) ;
#87004=CARTESIAN_POINT('',(79.2,253.900000000001,30.6213203435596)) ;
#87005=CARTESIAN_POINT('Origin',(79.1,253.900000000001,30.6213203435596)) ;
#87006=CARTESIAN_POINT('',(79.2,246.600000000001,30.6213203435596)) ;
#87007=CARTESIAN_POINT('Origin',(79.1,246.500000000001,30.6213203435596)) ;
#87008=CARTESIAN_POINT('',(79.2,246.138656108705,30.6213203435596)) ;
#87009=CARTESIAN_POINT('Origin',(79.2,253.900000000001,30.7213203435596)) ;
#87010=CARTESIAN_POINT('',(79.2,253.900000000001,30.7213203435596)) ;
#87011=CARTESIAN_POINT('',(79.2,246.600000000001,30.7213203435596)) ;
#87012=CARTESIAN_POINT('Origin',(83.6283628290597,244.119881553511,29.6213203435596)) ;
#87013=CARTESIAN_POINT('',(84.1283628290597,244.119881553511,29.6213203435596)) ;
#87014=CARTESIAN_POINT('Origin',(84.0283628290597,244.119881553511,29.6213203435596)) ;
#87015=CARTESIAN_POINT('',(84.0113850506192,244.441275358355,29.6213203435596)) ;
#87016=CARTESIAN_POINT('Origin',(83.9347806063073,244.376996597386,29.6213203435596)) ;
#87017=CARTESIAN_POINT('Origin',(83.6283628290597,244.119881553511,29.6213203435596)) ;
#87018=CARTESIAN_POINT('Origin',(83.6283628290597,244.119881553511,30.6213203435596)) ;
#87019=CARTESIAN_POINT('',(84.1283628290597,244.119881553511,30.6213203435596)) ;
#87020=CARTESIAN_POINT('Origin',(84.0283628290597,244.119881553511,30.6213203435596)) ;
#87021=CARTESIAN_POINT('',(84.0113850506192,244.441275358355,30.6213203435596)) ;
#87022=CARTESIAN_POINT('Origin',(83.6283628290597,244.119881553511,30.6213203435596)) ;
#87023=CARTESIAN_POINT('Origin',(83.9347806063073,244.376996597386,30.6213203435596)) ;
#87024=CARTESIAN_POINT('Origin',(83.6283628290597,244.119881553511,30.7213203435596)) ;
#87025=CARTESIAN_POINT('',(84.1283628290597,244.119881553511,30.7213203435596)) ;
#87026=CARTESIAN_POINT('',(84.0113850506192,244.441275358355,30.7213203435596)) ;
#87027=CARTESIAN_POINT('Origin',(84.1283628290597,244.301866670644,30.7213203435596)) ;
#87028=CARTESIAN_POINT('',(84.1283628290596,241.083851787777,30.6213203435596)) ;
#87029=CARTESIAN_POINT('',(84.1283628290597,241.339589444027,30.6213203435596)) ;
#87030=CARTESIAN_POINT('',(84.1283628290596,241.083851787777,29.6213203435596)) ;
#87031=CARTESIAN_POINT('',(84.1283628290597,241.083851787777,30.7213203435596)) ;
#87032=CARTESIAN_POINT('',(84.1283628290597,241.339589444027,29.6213203435596)) ;
#87033=CARTESIAN_POINT('Origin',(84.0283628290597,241.339589444027,30.6213203435596)) ;
#87034=CARTESIAN_POINT('Origin',(84.0283628290596,241.083851787777,30.6213203435596)) ;
#87035=CARTESIAN_POINT('Origin',(81.6097350811727,247.14787795491,30.6213203435596)) ;
#87036=CARTESIAN_POINT('',(82.349868392482,246.421393804845,30.6213203435596)) ;
#87037=CARTESIAN_POINT('',(81.6863395254846,247.212156715879,30.6213203435596)) ;
#87038=CARTESIAN_POINT('Origin',(82.2732639481701,246.357115043876,30.6213203435596)) ;
#87039=CARTESIAN_POINT('Origin',(81.9668461709225,246.100000000001,29.6213203435596)) ;
#87040=CARTESIAN_POINT('',(82.349868392482,246.421393804845,29.6213203435596)) ;
#87041=CARTESIAN_POINT('Origin',(82.2732639481701,246.357115043876,29.6213203435596)) ;
#87042=CARTESIAN_POINT('',(81.9668461709225,246.600000000001,29.6213203435596)) ;
#87043=CARTESIAN_POINT('Origin',(81.9668461709225,246.500000000001,29.6213203435596)) ;
#87044=CARTESIAN_POINT('Origin',(81.9668461709225,246.100000000001,29.6213203435596)) ;
#87045=CARTESIAN_POINT('Origin',(81.9668461709225,246.100000000001,30.6213203435596)) ;
#87046=CARTESIAN_POINT('',(81.9668461709225,246.600000000001,30.6213203435596)) ;
#87047=CARTESIAN_POINT('Origin',(81.9668461709225,246.100000000001,30.6213203435596)) ;
#87048=CARTESIAN_POINT('Origin',(81.9668461709225,246.500000000001,30.6213203435596)) ;
#87049=CARTESIAN_POINT('Origin',(81.9668461709225,246.100000000001,30.7213203435596)) ;
#87050=CARTESIAN_POINT('',(82.349868392482,246.421393804845,30.7213203435596)) ;
#87051=CARTESIAN_POINT('',(81.9668461709225,246.600000000001,30.7213203435596)) ;
#87052=CARTESIAN_POINT('Origin',(81.6097350811727,247.14787795491,29.6213203435596)) ;
#87053=CARTESIAN_POINT('',(81.6863395254846,247.212156715879,29.6213203435596)) ;
#87054=CARTESIAN_POINT('Origin',(82.2,246.600000000001,30.7213203435596)) ;
#87055=CARTESIAN_POINT('Origin',(83.6283628290597,241.083851787777,29.6213203435596)) ;
#87056=CARTESIAN_POINT('',(84.0113850506191,240.762457982934,29.6213203435596)) ;
#87057=CARTESIAN_POINT('Origin',(83.9347806063072,240.826736743903,29.6213203435596)) ;
#87058=CARTESIAN_POINT('Origin',(84.0283628290596,241.083851787777,29.6213203435596)) ;
#87059=CARTESIAN_POINT('Origin',(83.6283628290597,241.083851787777,29.6213203435596)) ;
#87060=CARTESIAN_POINT('Origin',(83.6283628290597,241.083851787777,30.6213203435596)) ;
#87061=CARTESIAN_POINT('',(84.0113850506191,240.762457982934,30.6213203435596)) ;
#87062=CARTESIAN_POINT('Origin',(83.9347806063072,240.826736743903,30.6213203435596)) ;
#87063=CARTESIAN_POINT('Origin',(83.6283628290597,241.083851787777,30.6213203435596)) ;
#87064=CARTESIAN_POINT('Origin',(83.6283628290597,241.083851787777,30.7213203435596)) ;
#87065=CARTESIAN_POINT('',(84.0113850506192,240.762457982934,30.7213203435596)) ;
#87066=CARTESIAN_POINT('Origin',(80.4937295064186,236.72585173331,29.6213203435596)) ;
#87067=CARTESIAN_POINT('',(82.2599473569929,238.67517581935,29.6213203435596)) ;
#87068=CARTESIAN_POINT('',(80.5703339507305,236.661572972341,29.6213203435596)) ;
#87069=CARTESIAN_POINT('Origin',(82.183342912681,238.739454580319,29.6213203435596)) ;
#87070=CARTESIAN_POINT('Origin',(84.1283628290597,240.901866670644,30.7213203435596)) ;
#87071=CARTESIAN_POINT('',(82.2599473569929,238.67517581935,30.6213203435596)) ;
#87072=CARTESIAN_POINT('',(80.5703339507305,236.661572972341,30.6213203435596)) ;
#87073=CARTESIAN_POINT('',(82.2599473569929,238.67517581935,30.7213203435596)) ;
#87074=CARTESIAN_POINT('Origin',(80.4937295064186,236.72585173331,30.6213203435596)) ;
#87075=CARTESIAN_POINT('Origin',(82.183342912681,238.739454580319,30.6213203435596)) ;
#87076=CARTESIAN_POINT('Ctrl Pts',(80.1000000000001,238.703733341287,30.7213203435596)) ;
#87077=CARTESIAN_POINT('Ctrl Pts',(80.1673349911517,238.681308542337,30.7213203435596)) ;
#87078=CARTESIAN_POINT('Ctrl Pts',(80.3246968018175,238.628902299152,30.70305597993)) ;
#87079=CARTESIAN_POINT('Ctrl Pts',(80.4001384593499,238.603722491233,30.6512500569856)) ;
#87080=CARTESIAN_POINT('Ctrl Pts',(80.4001060221343,238.603733317644,30.621286553673)) ;
#87081=CARTESIAN_POINT('Ctrl Pts',(80.1000000000001,238.703733341287,30.7213203435596)) ;
#87082=CARTESIAN_POINT('Ctrl Pts',(80.1598499591183,238.673823510303,30.7213203435596)) ;
#87083=CARTESIAN_POINT('Ctrl Pts',(80.3006804267155,238.603362191114,30.6841188443569)) ;
#87084=CARTESIAN_POINT('Ctrl Pts',(80.3477306429498,238.603762877822,30.635414869881)) ;
#87085=CARTESIAN_POINT('Ctrl Pts',(80.3477104110672,238.603762708834,30.6213044253022)) ;
#87086=CARTESIAN_POINT('Ctrl Pts',(80.1000000000001,238.703733341287,30.7213203435596)) ;
#87087=CARTESIAN_POINT('Ctrl Pts',(80.1448798950513,238.658853446236,30.7213203435596)) ;
#87088=CARTESIAN_POINT('Ctrl Pts',(80.2522646492235,238.551468692064,30.664890088409)) ;
#87089=CARTESIAN_POINT('Ctrl Pts',(80.2434889907335,238.560244350553,30.6174238570621)) ;
#87090=CARTESIAN_POINT('Ctrl Pts',(80.2434927581474,238.560240583139,30.6213247294469)) ;
#87091=CARTESIAN_POINT('Ctrl Pts',(80.1000000000001,238.703733341287,30.7213203435596)) ;
#87092=CARTESIAN_POINT('Ctrl Pts',(80.1299098309844,238.643883382169,30.7213203435596)) ;
#87093=CARTESIAN_POINT('Ctrl Pts',(80.2003711501734,238.503052914572,30.684118844357)) ;
#87094=CARTESIAN_POINT('Ctrl Pts',(80.1999704634652,238.456002698337,30.6354148698811)) ;
#87095=CARTESIAN_POINT('Ctrl Pts',(80.1999706324531,238.45602293022,30.6213044253022)) ;
#87096=CARTESIAN_POINT('Ctrl Pts',(80.1000000000001,238.703733341287,30.7213203435596)) ;
#87097=CARTESIAN_POINT('Ctrl Pts',(80.1224247989508,238.636398350136,30.7213203435596)) ;
#87098=CARTESIAN_POINT('Ctrl Pts',(80.1748310421352,238.479036539469,30.7030559799303)) ;
#87099=CARTESIAN_POINT('Ctrl Pts',(80.2000108500545,238.403594881936,30.6512500569859)) ;
#87100=CARTESIAN_POINT('Ctrl Pts',(80.2000000236427,238.403627319152,30.621286553673)) ;
#87101=CARTESIAN_POINT('',(80.2000000000001,238.403733341287,30.6213203435596)) ;
#87102=CARTESIAN_POINT('',(80.4000000000001,238.603733341287,30.6213203435596)) ;
#87103=CARTESIAN_POINT('Origin',(80.4000000000001,238.403733341287,30.6213203435596)) ;
#87104=CARTESIAN_POINT('',(80.2871000903541,238.641366644502,30.6994893600058)) ;
#87105=CARTESIAN_POINT('Origin',(80.1000000000001,238.703733341287,30.6213203435596)) ;
#87106=CARTESIAN_POINT('Origin',(80.1000000000001,238.703733341287,30.6213203435596)) ;
#87107=CARTESIAN_POINT('',(80.1623666967849,238.516633250933,30.6994893600057)) ;
#87108=CARTESIAN_POINT('Origin',(80.1000000000001,238.703733341287,30.6213203435596)) ;
#87109=CARTESIAN_POINT('Origin',(80.1000000000001,238.703733341287,30.6213203435596)) ;
#87110=CARTESIAN_POINT('Origin',(80.4000000000001,238.403733341287,30.7213203435596)) ;
#87111=CARTESIAN_POINT('',(80.2000000000001,238.403733341287,29.6213203435596)) ;
#87112=CARTESIAN_POINT('',(80.2000000000001,238.403733341287,30.7213203435596)) ;
#87113=CARTESIAN_POINT('',(80.4000000000001,238.603733341287,29.6213203435596)) ;
#87114=CARTESIAN_POINT('Origin',(80.4000000000001,238.403733341287,29.6213203435596)) ;
#87115=CARTESIAN_POINT('',(80.4000000000001,238.603733341287,30.7213203435596)) ;
#87116=CARTESIAN_POINT('Ctrl Pts',(80.1000000000001,238.703733341287,29.5213203435596)) ;
#87117=CARTESIAN_POINT('Ctrl Pts',(80.12242479571,238.636398346894,29.5213203435596)) ;
#87118=CARTESIAN_POINT('Ctrl Pts',(80.1748310522054,238.479036465714,29.539584677183)) ;
#87119=CARTESIAN_POINT('Ctrl Pts',(80.2000108523797,238.40359485233,29.5913906280511)) ;
#87120=CARTESIAN_POINT('Ctrl Pts',(80.2000000236528,238.403627296473,29.6213541406864)) ;
#87121=CARTESIAN_POINT('Ctrl Pts',(80.1000000000001,238.703733341287,29.5213203435596)) ;
#87122=CARTESIAN_POINT('Ctrl Pts',(80.1299098288238,238.643883380009,29.5213203435596)) ;
#87123=CARTESIAN_POINT('Ctrl Pts',(80.2003711613395,238.503052837057,29.5585219149689)) ;
#87124=CARTESIAN_POINT('Ctrl Pts',(80.1999704571707,238.456002678962,29.6072258190892)) ;
#87125=CARTESIAN_POINT('Ctrl Pts',(80.1999706262014,238.456022915153,29.6213362652259)) ;
#87126=CARTESIAN_POINT('Ctrl Pts',(80.1000000000001,238.703733341287,29.5213203435596)) ;
#87127=CARTESIAN_POINT('Ctrl Pts',(80.1448798950518,238.658853446236,29.5213203435596)) ;
#87128=CARTESIAN_POINT('Ctrl Pts',(80.2522647587334,238.551468582557,29.5777508728895)) ;
#87129=CARTESIAN_POINT('Ctrl Pts',(80.2434889412482,238.560244400044,29.6252168369043)) ;
#87130=CARTESIAN_POINT('Ctrl Pts',(80.2434927095359,238.560240631756,29.6213159567278)) ;
#87131=CARTESIAN_POINT('Ctrl Pts',(80.1000000000001,238.703733341287,29.5213203435596)) ;
#87132=CARTESIAN_POINT('Ctrl Pts',(80.15984996128,238.673823512465,29.5213203435596)) ;
#87133=CARTESIAN_POINT('Ctrl Pts',(80.300680504234,238.603362179951,29.5585219149676)) ;
#87134=CARTESIAN_POINT('Ctrl Pts',(80.3477306623321,238.603762884119,29.607225819088)) ;
#87135=CARTESIAN_POINT('Ctrl Pts',(80.3477104261414,238.603762715089,29.6213362652259)) ;
#87136=CARTESIAN_POINT('Ctrl Pts',(80.1000000000001,238.703733341287,29.5213203435596)) ;
#87137=CARTESIAN_POINT('Ctrl Pts',(80.1673349943943,238.681308545579,29.5213203435596)) ;
#87138=CARTESIAN_POINT('Ctrl Pts',(80.3246968755785,238.628902289088,29.5395846771792)) ;
#87139=CARTESIAN_POINT('Ctrl Pts',(80.4001384889675,238.603722488907,29.5913906280479)) ;
#87140=CARTESIAN_POINT('Ctrl Pts',(80.4001060448247,238.603733317634,29.6213541406864)) ;
#87141=CARTESIAN_POINT('',(80.1623667045681,238.516633227583,29.5431513333233)) ;
#87142=CARTESIAN_POINT('Origin',(80.1000000000001,238.703733341287,29.6213203435596)) ;
#87143=CARTESIAN_POINT('Origin',(80.1000000000001,238.703733341287,29.6213203435596)) ;
#87144=CARTESIAN_POINT('',(80.2871001137062,238.641366636718,29.5431513333238)) ;
#87145=CARTESIAN_POINT('Origin',(80.1000000000001,238.703733341287,29.6213203435596)) ;
#87146=CARTESIAN_POINT('Origin',(80.1000000000001,238.703733341287,29.6213203435596)) ;
#87147=CARTESIAN_POINT('Origin',(80.2000000000001,238.603733341287,30.7213203435596)) ;
#87148=CARTESIAN_POINT('',(80.2000000000001,235.603733341287,30.6213203435596)) ;
#87149=CARTESIAN_POINT('',(80.2000000000001,238.490522779348,30.6213203435596)) ;
#87150=CARTESIAN_POINT('',(80.2000000000001,235.603733341287,29.6213203435596)) ;
#87151=CARTESIAN_POINT('',(80.2000000000001,235.603733341287,30.7213203435596)) ;
#87152=CARTESIAN_POINT('',(80.2000000000001,238.490522779348,29.6213203435596)) ;
#87153=CARTESIAN_POINT('Origin',(80.1000000000001,238.490522779348,30.6213203435596)) ;
#87154=CARTESIAN_POINT('Origin',(80.1000000000001,235.614468918958,30.6213203435596)) ;
#87155=CARTESIAN_POINT('Origin',(76.057090707265,238.703733341287,30.6213203435596)) ;
#87156=CARTESIAN_POINT('',(82.1067384683691,238.603733341287,30.6213203435596)) ;
#87157=CARTESIAN_POINT('',(76.057090707265,238.603733341287,30.6213203435596)) ;
#87158=CARTESIAN_POINT('Origin',(82.1067384683691,238.703733341287,30.6213203435596)) ;
#87159=CARTESIAN_POINT('Ctrl Pts',(82.2599473569933,238.67517581935,29.6213203435597)) ;
#87160=CARTESIAN_POINT('Ctrl Pts',(82.1999999999999,238.603733341287,29.6213203435598)) ;
#87161=CARTESIAN_POINT('Ctrl Pts',(82.106738468368,238.603733341287,29.6213203435596)) ;
#87162=CARTESIAN_POINT('Ctrl Pts',(82.2599473569934,238.67517581935,29.5213203435594)) ;
#87163=CARTESIAN_POINT('Ctrl Pts',(82.2,238.603733341287,29.5213203435595)) ;
#87164=CARTESIAN_POINT('Ctrl Pts',(82.1067384683682,238.603733341287,29.5213203435592)) ;
#87165=CARTESIAN_POINT('Ctrl Pts',(82.183342912681,238.739454580319,29.5213203435596)) ;
#87166=CARTESIAN_POINT('Ctrl Pts',(82.1533692341843,238.703733341287,29.5213203435597)) ;
#87167=CARTESIAN_POINT('Ctrl Pts',(82.1067384683682,238.703733341287,29.5213203435596)) ;
#87168=CARTESIAN_POINT('',(82.1067384683691,238.603733341287,29.6213203435596)) ;
#87169=CARTESIAN_POINT('Origin',(82.1067384683691,238.703733341287,29.6213203435596)) ;
#87170=CARTESIAN_POINT('Origin',(82.1067384683691,238.803733341287,29.6213203435596)) ;
#87171=CARTESIAN_POINT('Ctrl Pts',(82.183342912681,238.739454580319,30.7213203435596)) ;
#87172=CARTESIAN_POINT('Ctrl Pts',(82.1533692341851,238.703733341287,30.7213203435595)) ;
#87173=CARTESIAN_POINT('Ctrl Pts',(82.1067384683691,238.703733341287,30.7213203435597)) ;
#87174=CARTESIAN_POINT('Ctrl Pts',(82.2599473569944,238.675175819352,30.7213203435596)) ;
#87175=CARTESIAN_POINT('Ctrl Pts',(82.2000000000015,238.603733341286,30.7213203435595)) ;
#87176=CARTESIAN_POINT('Ctrl Pts',(82.1067384683677,238.603733341287,30.7213203435597)) ;
#87177=CARTESIAN_POINT('Ctrl Pts',(82.2599473569945,238.675175819352,30.6213203435595)) ;
#87178=CARTESIAN_POINT('Ctrl Pts',(82.2000000000014,238.603733341286,30.6213203435594)) ;
#87179=CARTESIAN_POINT('Ctrl Pts',(82.1067384683674,238.603733341287,30.6213203435596)) ;
#87180=CARTESIAN_POINT('Origin',(82.1067384683691,238.803733341287,30.6213203435596)) ;
#87181=CARTESIAN_POINT('Origin',(82.1067384683691,238.803733341287,30.7213203435596)) ;
#87182=CARTESIAN_POINT('',(82.1067384683691,238.603733341287,30.7213203435596)) ;
#87183=CARTESIAN_POINT('Origin',(76.057090707265,238.703733341287,29.6213203435596)) ;
#87184=CARTESIAN_POINT('',(76.057090707265,238.603733341287,29.6213203435596)) ;
#87185=CARTESIAN_POINT('Origin',(82.2000000000001,238.603733341287,30.7213203435596)) ;
#87186=CARTESIAN_POINT('Origin',(75.3756995384723,240.638656108705,30.6213203435596)) ;
#87187=CARTESIAN_POINT('',(75.4756995384723,242.900000000001,30.6213203435596)) ;
#87188=CARTESIAN_POINT('Origin',(75.3756995384723,242.900000000001,30.6213203435596)) ;
#87189=CARTESIAN_POINT('',(75.4756995384723,240.900000000001,30.6213203435596)) ;
#87190=CARTESIAN_POINT('Origin',(75.3756995384723,240.900000000001,30.6213203435596)) ;
#87191=CARTESIAN_POINT('',(75.4756995384723,240.638656108705,30.6213203435596)) ;
#87192=CARTESIAN_POINT('Origin',(76.9283628290597,240.900000000001,30.6213203435596)) ;
#87193=CARTESIAN_POINT('',(78.381026119647,240.900000000001,30.6213203435596)) ;
#87194=CARTESIAN_POINT('Origin',(78.481026119647,240.900000000001,30.6213203435596)) ;
#87195=CARTESIAN_POINT('Origin',(76.9283628290597,240.900000000001,30.6213203435596)) ;
#87196=CARTESIAN_POINT('Origin',(78.481026119647,239.638656108705,30.6213203435596)) ;
#87197=CARTESIAN_POINT('',(78.381026119647,242.900000000001,30.6213203435596)) ;
#87198=CARTESIAN_POINT('Origin',(78.481026119647,242.900000000001,30.6213203435596)) ;
#87199=CARTESIAN_POINT('',(78.381026119647,239.638656108705,30.6213203435596)) ;
#87200=CARTESIAN_POINT('Origin',(76.9283628290597,242.900000000001,30.6213203435596)) ;
#87201=CARTESIAN_POINT('Origin',(76.9283628290597,242.900000000001,30.6213203435596)) ;
#87202=CARTESIAN_POINT('Origin',(76.9283628290597,242.900000000001,30.7213203435596)) ;
#87203=CARTESIAN_POINT('',(75.4756995384723,242.900000000001,30.7213203435596)) ;
#87204=CARTESIAN_POINT('',(78.381026119647,242.900000000001,30.7213203435596)) ;
#87205=CARTESIAN_POINT('Origin',(75.4756995384723,242.900000000001,30.7213203435596)) ;
#87206=CARTESIAN_POINT('',(75.4756995384723,240.900000000001,30.7213203435596)) ;
#87207=CARTESIAN_POINT('Origin',(75.1450953968556,223.000000000001,30.6213203435596)) ;
#87208=CARTESIAN_POINT('',(74.7,226.000000000001,30.6954104575527)) ;
#87209=CARTESIAN_POINT('Ctrl Pts',(74.7,226.000000000001,30.6954104575527)) ;
#87210=CARTESIAN_POINT('Ctrl Pts',(74.7,226.008355406754,30.7029024804683)) ;
#87211=CARTESIAN_POINT('Ctrl Pts',(74.7,226.019099007153,30.709548142939)) ;
#87212=CARTESIAN_POINT('Ctrl Pts',(74.7,226.040633652905,30.7184120613473)) ;
#87213=CARTESIAN_POINT('Ctrl Pts',(74.7,226.055366277592,30.7213203435596)) ;
#87214=CARTESIAN_POINT('Ctrl Pts',(74.7,226.067880390058,30.7213203435596)) ;
#87215=CARTESIAN_POINT('',(75.1450953968557,226.000000000001,30.6213203435596)) ;
#87216=CARTESIAN_POINT('Origin',(75.1450953968556,223.000000000001,30.6213203435596)) ;
#87217=CARTESIAN_POINT('Ctrl Pts',(75.1450953968556,226.000000000001,30.6213203435596)) ;
#87218=CARTESIAN_POINT('Ctrl Pts',(75.0066828077914,226.000000000001,30.6465909093173)) ;
#87219=CARTESIAN_POINT('Ctrl Pts',(74.8525909945362,226.000000000001,30.6751106345129)) ;
#87220=CARTESIAN_POINT('Ctrl Pts',(74.7,226.000000000001,30.6954104575527)) ;
#87221=CARTESIAN_POINT('Origin',(74.7,226.000000000001,30.7213203435596)) ;
#87222=CARTESIAN_POINT('',(75.1450953968557,226.000000000001,29.6213203435596)) ;
#87223=CARTESIAN_POINT('',(75.1450953968557,226.000000000001,30.7213203435596)) ;
#87224=CARTESIAN_POINT('',(74.7,226.000000000001,29.5472302295665)) ;
#87225=CARTESIAN_POINT('Ctrl Pts',(74.7,226.000000000001,29.5472302295665)) ;
#87226=CARTESIAN_POINT('Ctrl Pts',(74.8525909945361,226.000000000001,29.5675300526063)) ;
#87227=CARTESIAN_POINT('Ctrl Pts',(75.0066828077914,226.000000000001,29.5960497778019)) ;
#87228=CARTESIAN_POINT('Ctrl Pts',(75.1450953968556,226.000000000001,29.6213203435596)) ;
#87229=CARTESIAN_POINT('',(74.7,226.000000000001,30.7213203435596)) ;
#87230=CARTESIAN_POINT('Origin',(75.1450953968556,223.000000000001,30.7213203435596)) ;
#87231=CARTESIAN_POINT('Origin',(75.1450953968556,223.000000000001,29.6213203435596)) ;
#87232=CARTESIAN_POINT('Origin',(72.1450953968557,220.362610236549,30.7213203435596)) ;
#87233=CARTESIAN_POINT('',(66.5470607720161,220.362610236549,30.7213203435596)) ;
#87234=CARTESIAN_POINT('Origin',(75.1450953968556,223.000000000001,29.6213203435596)) ;
#87235=CARTESIAN_POINT('Ctrl Pts',(74.7,226.067880390058,29.5213203435596)) ;
#87236=CARTESIAN_POINT('Ctrl Pts',(74.7,226.055366277592,29.5213203435595)) ;
#87237=CARTESIAN_POINT('Ctrl Pts',(74.7,226.040633652905,29.5242286257719)) ;
#87238=CARTESIAN_POINT('Ctrl Pts',(74.7,226.019099007153,29.5330925441802)) ;
#87239=CARTESIAN_POINT('Ctrl Pts',(74.7,226.008355406754,29.5397382066508)) ;
#87240=CARTESIAN_POINT('Ctrl Pts',(74.7,226.000000000001,29.5472302295665)) ;
#87241=CARTESIAN_POINT('Origin',(74.7,231.000000000001,30.7213203435596)) ;
#87242=CARTESIAN_POINT('',(74.7,231.000000000001,30.7213203435596)) ;
#87243=CARTESIAN_POINT('Origin',(80.1582163984138,235.882481693345,29.6213203435596)) ;
#87244=CARTESIAN_POINT('',(79.2,231.000000000001,29.6213203435596)) ;
#87245=CARTESIAN_POINT('',(80.2559376094964,235.861255179157,29.6213203435596)) ;
#87246=CARTESIAN_POINT('Origin',(79.0976680713511,231.000000000001,29.6213203435596)) ;
#87247=CARTESIAN_POINT('Origin',(80.1000000000001,235.614468918958,29.6213203435596)) ;
#87248=CARTESIAN_POINT('Origin',(80.1000000000001,238.490522779348,29.6213203435596)) ;
#87249=CARTESIAN_POINT('Origin',(84.0283628290597,241.339589444027,29.6213203435596)) ;
#87250=CARTESIAN_POINT('Origin',(74.5570907072649,246.500000000001,29.6213203435596)) ;
#87251=CARTESIAN_POINT('',(74.5570907072649,246.600000000001,29.6213203435596)) ;
#87252=CARTESIAN_POINT('Origin',(79.2,231.000000000001,30.7213203435596)) ;
#87253=CARTESIAN_POINT('',(79.2,231.000000000001,30.6213203435596)) ;
#87254=CARTESIAN_POINT('',(79.2,231.000000000001,30.7213203435596)) ;
#87255=CARTESIAN_POINT('Origin',(79.0976680713511,231.000000000001,30.6213203435596)) ;
#87256=CARTESIAN_POINT('Origin',(80.2000000000001,235.603733341287,30.7213203435596)) ;
#87257=CARTESIAN_POINT('',(80.2559376094964,235.861255179157,30.6213203435596)) ;
#87258=CARTESIAN_POINT('Origin',(79.2,246.600000000001,30.7213203435596)) ;
#87259=CARTESIAN_POINT('',(74.5570907072649,246.600000000001,30.6213203435596)) ;
#87260=CARTESIAN_POINT('Origin',(74.5570907072649,246.500000000001,30.6213203435596)) ;
#87261=CARTESIAN_POINT('Origin',(80.1582163984138,235.882481693345,30.6213203435596)) ;
#87262=CARTESIAN_POINT('Origin',(57.,255.80417392569,30.6213203435596)) ;
#87263=CARTESIAN_POINT('',(56.7,255.80417392569,31.5213203435596)) ;
#87264=CARTESIAN_POINT('',(57.,255.80417392569,31.8213203435596)) ;
#87265=CARTESIAN_POINT('Origin',(57.,255.80417392569,31.5213203435596)) ;
#87266=CARTESIAN_POINT('Origin',(57.,255.80417392569,30.6213203435596)) ;
#87267=CARTESIAN_POINT('Origin',(56.7,255.80417392569,30.6213203435596)) ;
#87268=CARTESIAN_POINT('Origin',(57.,256.4,31.5213203435596)) ;
#87269=CARTESIAN_POINT('',(56.7,255.79582607431,31.5213203435596)) ;
#87270=CARTESIAN_POINT('',(57.,255.79582607431,31.8213203435596)) ;
#87271=CARTESIAN_POINT('Origin',(57.,255.79582607431,31.5213203435596)) ;
#87272=CARTESIAN_POINT('',(57.,256.4,31.8213203435596)) ;
#87273=CARTESIAN_POINT('',(56.7,256.4,31.5213203435596)) ;
#87274=CARTESIAN_POINT('Origin',(57.,255.79582607431,30.6213203435596)) ;
#87275=CARTESIAN_POINT('Origin',(57.,255.79582607431,30.6213203435596)) ;
#87276=CARTESIAN_POINT('Origin',(56.7,255.79582607431,30.6213203435596)) ;
#87277=CARTESIAN_POINT('Origin',(56.7,257.,30.2213203435596)) ;
#87278=CARTESIAN_POINT('Origin',(58.8,255.79582607431,30.6213203435596)) ;
#87279=CARTESIAN_POINT('',(59.1,255.79582607431,31.5213203435596)) ;
#87280=CARTESIAN_POINT('',(58.8,255.79582607431,31.8213203435596)) ;
#87281=CARTESIAN_POINT('Origin',(58.8,255.79582607431,31.5213203435596)) ;
#87282=CARTESIAN_POINT('Origin',(58.8,255.79582607431,30.6213203435596)) ;
#87283=CARTESIAN_POINT('Origin',(59.1,255.79582607431,30.6213203435596)) ;
#87284=CARTESIAN_POINT('Origin',(58.8,255.2,31.5213203435596)) ;
#87285=CARTESIAN_POINT('',(59.1,255.80417392569,31.5213203435596)) ;
#87286=CARTESIAN_POINT('',(58.8,255.80417392569,31.8213203435596)) ;
#87287=CARTESIAN_POINT('Origin',(58.8,255.80417392569,31.5213203435596)) ;
#87288=CARTESIAN_POINT('',(58.8,255.2,31.8213203435596)) ;
#87289=CARTESIAN_POINT('',(59.1,255.2,31.5213203435596)) ;
#87290=CARTESIAN_POINT('Origin',(58.8,255.80417392569,30.6213203435596)) ;
#87291=CARTESIAN_POINT('Origin',(58.8,255.80417392569,30.6213203435596)) ;
#87292=CARTESIAN_POINT('Origin',(59.1,255.80417392569,30.6213203435596)) ;
#87293=CARTESIAN_POINT('Origin',(59.1,254.6,30.2213203435596)) ;
#87294=CARTESIAN_POINT('Origin',(66.8,255.79582607431,30.6213203435596)) ;
#87295=CARTESIAN_POINT('',(67.1,255.79582607431,31.5213203435596)) ;
#87296=CARTESIAN_POINT('',(66.8,255.79582607431,31.8213203435596)) ;
#87297=CARTESIAN_POINT('Origin',(66.8,255.79582607431,31.5213203435596)) ;
#87298=CARTESIAN_POINT('Origin',(66.8,255.79582607431,30.6213203435596)) ;
#87299=CARTESIAN_POINT('Origin',(67.1,255.79582607431,30.6213203435596)) ;
#87300=CARTESIAN_POINT('Origin',(66.8,255.2,31.5213203435596)) ;
#87301=CARTESIAN_POINT('',(67.1,255.80417392569,31.5213203435596)) ;
#87302=CARTESIAN_POINT('',(66.8,255.80417392569,31.8213203435596)) ;
#87303=CARTESIAN_POINT('Origin',(66.8,255.80417392569,31.5213203435596)) ;
#87304=CARTESIAN_POINT('',(66.8,255.2,31.8213203435596)) ;
#87305=CARTESIAN_POINT('',(67.1,255.2,31.5213203435596)) ;
#87306=CARTESIAN_POINT('Origin',(66.8,255.80417392569,30.6213203435596)) ;
#87307=CARTESIAN_POINT('Origin',(66.8,255.80417392569,30.6213203435596)) ;
#87308=CARTESIAN_POINT('Origin',(67.1,255.80417392569,30.6213203435596)) ;
#87309=CARTESIAN_POINT('Origin',(67.1,254.6,30.2213203435596)) ;
#87310=CARTESIAN_POINT('Origin',(65.,255.80417392569,30.6213203435596)) ;
#87311=CARTESIAN_POINT('',(64.7,255.80417392569,31.5213203435596)) ;
#87312=CARTESIAN_POINT('',(65.,255.80417392569,31.8213203435596)) ;
#87313=CARTESIAN_POINT('Origin',(65.,255.80417392569,31.5213203435596)) ;
#87314=CARTESIAN_POINT('Origin',(65.,255.80417392569,30.6213203435596)) ;
#87315=CARTESIAN_POINT('Origin',(64.7,255.80417392569,30.6213203435596)) ;
#87316=CARTESIAN_POINT('Origin',(65.,256.4,31.5213203435596)) ;
#87317=CARTESIAN_POINT('',(64.7,255.79582607431,31.5213203435596)) ;
#87318=CARTESIAN_POINT('',(65.,255.79582607431,31.8213203435596)) ;
#87319=CARTESIAN_POINT('Origin',(65.,255.79582607431,31.5213203435596)) ;
#87320=CARTESIAN_POINT('',(65.,256.4,31.8213203435596)) ;
#87321=CARTESIAN_POINT('',(64.7,256.4,31.5213203435596)) ;
#87322=CARTESIAN_POINT('Origin',(65.,255.79582607431,30.6213203435596)) ;
#87323=CARTESIAN_POINT('Origin',(65.,255.79582607431,30.6213203435596)) ;
#87324=CARTESIAN_POINT('Origin',(64.7,255.79582607431,30.6213203435596)) ;
#87325=CARTESIAN_POINT('Origin',(64.7,257.,30.2213203435596)) ;
#87326=CARTESIAN_POINT('Origin',(62.0573593128807,234.79582607431,30.6213203435596)) ;
#87327=CARTESIAN_POINT('',(62.3573593128808,234.79582607431,31.5213203435596)) ;
#87328=CARTESIAN_POINT('',(62.0573593128807,234.79582607431,31.8213203435596)) ;
#87329=CARTESIAN_POINT('Origin',(62.0573593128807,234.79582607431,31.5213203435596)) ;
#87330=CARTESIAN_POINT('Origin',(62.0573593128807,234.79582607431,30.6213203435596)) ;
#87331=CARTESIAN_POINT('Origin',(62.3573593128808,234.79582607431,30.6213203435596)) ;
#87332=CARTESIAN_POINT('Origin',(62.0573593128807,234.2,31.5213203435596)) ;
#87333=CARTESIAN_POINT('',(62.3573593128808,234.80417392569,31.5213203435596)) ;
#87334=CARTESIAN_POINT('',(62.0573593128807,234.80417392569,31.8213203435596)) ;
#87335=CARTESIAN_POINT('Origin',(62.0573593128807,234.80417392569,31.5213203435596)) ;
#87336=CARTESIAN_POINT('',(62.0573593128807,234.2,31.8213203435596)) ;
#87337=CARTESIAN_POINT('',(62.3573593128808,234.2,31.5213203435596)) ;
#87338=CARTESIAN_POINT('Origin',(62.0573593128807,234.80417392569,30.6213203435596)) ;
#87339=CARTESIAN_POINT('Origin',(62.0573593128807,234.80417392569,30.6213203435596)) ;
#87340=CARTESIAN_POINT('Origin',(62.3573593128808,234.80417392569,30.6213203435596)) ;
#87341=CARTESIAN_POINT('Origin',(62.3573593128808,233.6,30.2213203435596)) ;
#87342=CARTESIAN_POINT('Origin',(60.2573593128808,234.80417392569,30.6213203435596)) ;
#87343=CARTESIAN_POINT('',(59.9573593128807,234.80417392569,31.5213203435596)) ;
#87344=CARTESIAN_POINT('',(60.2573593128808,234.80417392569,31.8213203435596)) ;
#87345=CARTESIAN_POINT('Origin',(60.2573593128808,234.80417392569,31.5213203435596)) ;
#87346=CARTESIAN_POINT('Origin',(60.2573593128808,234.80417392569,30.6213203435596)) ;
#87347=CARTESIAN_POINT('Origin',(59.9573593128807,234.80417392569,30.6213203435596)) ;
#87348=CARTESIAN_POINT('Origin',(60.2573593128808,235.4,31.5213203435596)) ;
#87349=CARTESIAN_POINT('',(59.9573593128807,234.79582607431,31.5213203435596)) ;
#87350=CARTESIAN_POINT('',(60.2573593128808,234.79582607431,31.8213203435596)) ;
#87351=CARTESIAN_POINT('Origin',(60.2573593128808,234.79582607431,31.5213203435596)) ;
#87352=CARTESIAN_POINT('',(60.2573593128808,235.4,31.8213203435596)) ;
#87353=CARTESIAN_POINT('',(59.9573593128807,235.4,31.5213203435596)) ;
#87354=CARTESIAN_POINT('Origin',(60.2573593128808,234.79582607431,30.6213203435596)) ;
#87355=CARTESIAN_POINT('Origin',(60.2573593128808,234.79582607431,30.6213203435596)) ;
#87356=CARTESIAN_POINT('Origin',(59.9573593128807,234.79582607431,30.6213203435596)) ;
#87357=CARTESIAN_POINT('Origin',(59.9573593128807,236.,30.2213203435596)) ;
#87358=CARTESIAN_POINT('Origin',(73.9,230.79582607431,30.6213203435596)) ;
#87359=CARTESIAN_POINT('',(74.2,230.79582607431,31.5213203435596)) ;
#87360=CARTESIAN_POINT('',(73.9,230.79582607431,31.8213203435596)) ;
#87361=CARTESIAN_POINT('Origin',(73.9,230.79582607431,31.5213203435596)) ;
#87362=CARTESIAN_POINT('Origin',(73.9,230.79582607431,30.6213203435596)) ;
#87363=CARTESIAN_POINT('Origin',(74.2,230.79582607431,30.6213203435596)) ;
#87364=CARTESIAN_POINT('Origin',(73.9,230.2,31.5213203435596)) ;
#87365=CARTESIAN_POINT('',(74.2,230.80417392569,31.5213203435596)) ;
#87366=CARTESIAN_POINT('',(73.9,230.80417392569,31.8213203435596)) ;
#87367=CARTESIAN_POINT('Origin',(73.9,230.80417392569,31.5213203435596)) ;
#87368=CARTESIAN_POINT('',(73.9,230.2,31.8213203435596)) ;
#87369=CARTESIAN_POINT('',(74.2,230.2,31.5213203435596)) ;
#87370=CARTESIAN_POINT('Origin',(73.9,230.80417392569,30.6213203435596)) ;
#87371=CARTESIAN_POINT('Origin',(73.9,230.80417392569,30.6213203435596)) ;
#87372=CARTESIAN_POINT('Origin',(74.2,230.80417392569,30.6213203435596)) ;
#87373=CARTESIAN_POINT('Origin',(74.2,229.6,30.2213203435596)) ;
#87374=CARTESIAN_POINT('Origin',(72.1,230.80417392569,30.6213203435596)) ;
#87375=CARTESIAN_POINT('',(71.8,230.80417392569,31.5213203435596)) ;
#87376=CARTESIAN_POINT('',(72.1,230.80417392569,31.8213203435596)) ;
#87377=CARTESIAN_POINT('Origin',(72.1,230.80417392569,31.5213203435596)) ;
#87378=CARTESIAN_POINT('Origin',(72.1,230.80417392569,30.6213203435596)) ;
#87379=CARTESIAN_POINT('Origin',(71.8,230.80417392569,30.6213203435596)) ;
#87380=CARTESIAN_POINT('Origin',(72.1,231.4,31.5213203435596)) ;
#87381=CARTESIAN_POINT('',(71.8,230.79582607431,31.5213203435596)) ;
#87382=CARTESIAN_POINT('',(72.1,230.79582607431,31.8213203435596)) ;
#87383=CARTESIAN_POINT('Origin',(72.1,230.79582607431,31.5213203435596)) ;
#87384=CARTESIAN_POINT('',(72.1,231.4,31.8213203435596)) ;
#87385=CARTESIAN_POINT('',(71.8,231.4,31.5213203435596)) ;
#87386=CARTESIAN_POINT('Origin',(72.1,230.79582607431,30.6213203435596)) ;
#87387=CARTESIAN_POINT('Origin',(72.1,230.79582607431,30.6213203435596)) ;
#87388=CARTESIAN_POINT('Origin',(71.8,230.79582607431,30.6213203435596)) ;
#87389=CARTESIAN_POINT('Origin',(71.8,232.,30.2213203435596)) ;
#87390=CARTESIAN_POINT('Origin',(71.8,230.80417392569,30.6213203435596)) ;
#87391=CARTESIAN_POINT('',(71.8,230.80417392569,31.8213203435596)) ;
#87392=CARTESIAN_POINT('Origin',(73.,230.8,31.8213203435596)) ;
#87393=CARTESIAN_POINT('',(74.2,230.79582607431,31.8213203435596)) ;
#87394=CARTESIAN_POINT('Origin',(74.2,230.79582607431,30.6213203435596)) ;
#87395=CARTESIAN_POINT('Origin',(66.1357703637053,234.80417392569,30.6213203435596)) ;
#87396=CARTESIAN_POINT('',(66.1357703637053,234.80417392569,31.8213203435596)) ;
#87397=CARTESIAN_POINT('Origin',(61.1573593128808,234.8,31.8213203435596)) ;
#87398=CARTESIAN_POINT('',(64.9357703637053,234.79582607431,31.8213203435596)) ;
#87399=CARTESIAN_POINT('Origin',(64.9357703637053,234.79582607431,30.6213203435596)) ;
#87400=CARTESIAN_POINT('Origin',(67.3070907072649,255.79582607431,30.6213203435596)) ;
#87401=CARTESIAN_POINT('',(67.3070907072649,255.79582607431,31.8213203435596)) ;
#87402=CARTESIAN_POINT('Origin',(65.9,255.8,31.8213203435596)) ;
#87403=CARTESIAN_POINT('',(68.5070907072649,255.80417392569,31.8213203435596)) ;
#87404=CARTESIAN_POINT('Origin',(68.5070907072649,255.80417392569,30.6213203435596)) ;
#87405=CARTESIAN_POINT('Origin',(64.5070907072649,255.80417392569,30.6213203435596)) ;
#87406=CARTESIAN_POINT('',(64.5070907072649,255.80417392569,31.8213203435596)) ;
#87407=CARTESIAN_POINT('Origin',(57.9,255.8,31.8213203435596)) ;
#87408=CARTESIAN_POINT('',(63.3070907072649,255.79582607431,31.8213203435596)) ;
#87409=CARTESIAN_POINT('Origin',(63.3070907072649,255.79582607431,30.6213203435596)) ;
#87410=CARTESIAN_POINT('Origin',(73.,230.8,30.2213203435596)) ;
#87411=CARTESIAN_POINT('',(74.2,229.6,30.2213203435596)) ;
#87412=CARTESIAN_POINT('',(74.2,232.,30.2213203435596)) ;
#87413=CARTESIAN_POINT('',(74.2,230.2,30.2213203435596)) ;
#87414=CARTESIAN_POINT('',(71.8,229.6,30.2213203435596)) ;
#87415=CARTESIAN_POINT('',(72.4,229.6,30.2213203435596)) ;
#87416=CARTESIAN_POINT('',(71.8,232.,30.2213203435596)) ;
#87417=CARTESIAN_POINT('',(71.8,231.4,30.2213203435596)) ;
#87418=CARTESIAN_POINT('',(73.6,232.,30.2213203435596)) ;
#87419=CARTESIAN_POINT('Origin',(74.2,232.,30.7213203435596)) ;
#87420=CARTESIAN_POINT('',(71.8,232.,30.7213203435596)) ;
#87421=CARTESIAN_POINT('',(74.2,232.,30.7213203435596)) ;
#87422=CARTESIAN_POINT('Origin',(71.8,232.,30.7213203435596)) ;
#87423=CARTESIAN_POINT('',(71.8,229.6,30.7213203435596)) ;
#87424=CARTESIAN_POINT('Origin',(64.1568347953872,220.146231446812,30.7213203435596)) ;
#87425=CARTESIAN_POINT('',(61.775147916658,220.442149698512,30.7213203435596)) ;
#87426=CARTESIAN_POINT('Origin',(62.3665731005048,219.254624434818,30.7213203435596)) ;
#87427=CARTESIAN_POINT('',(58.9573593128807,226.1,30.7213203435596)) ;
#87428=CARTESIAN_POINT('Origin',(78.381026119647,240.900000000001,30.7213203435596)) ;
#87429=CARTESIAN_POINT('',(78.381026119647,240.900000000001,30.7213203435596)) ;
#87430=CARTESIAN_POINT('Origin',(76.9283628290597,240.900000000001,30.7213203435596)) ;
#87431=CARTESIAN_POINT('Origin',(71.8,229.6,30.7213203435596)) ;
#87432=CARTESIAN_POINT('',(74.2,229.6,30.7213203435596)) ;
#87433=CARTESIAN_POINT('Origin',(74.2,229.6,30.7213203435596)) ;
#87434=CARTESIAN_POINT('Origin',(67.6,253.900000000001,30.7213203435596)) ;
#87435=CARTESIAN_POINT('',(67.6,253.900000000001,30.7213203435596)) ;
#87436=CARTESIAN_POINT('Origin',(67.6,257.5,30.7213203435596)) ;
#87437=CARTESIAN_POINT('',(67.6,257.5,30.7213203435596)) ;
#87438=CARTESIAN_POINT('Origin',(55.7,257.5,30.7213203435596)) ;
#87439=CARTESIAN_POINT('',(55.7,257.5,30.7213203435596)) ;
#87440=CARTESIAN_POINT('Origin',(55.7,245.9,30.7213203435596)) ;
#87441=CARTESIAN_POINT('',(55.7,245.9,30.7213203435596)) ;
#87442=CARTESIAN_POINT('Origin',(58.9573593128807,245.9,30.7213203435596)) ;
#87443=CARTESIAN_POINT('',(58.9573593128807,245.9,30.7213203435596)) ;
#87444=CARTESIAN_POINT('Origin',(58.9573593128807,226.1,30.7213203435596)) ;
#117130=UNCERTAINTY_MEASURE_WITH_UNIT(LENGTH_MEASURE(0.01),#117171,
'DISTANCE_ACCURACY_VALUE',
'Maximum model space distance between geometric entities at asserted c
onnectivities') ;
#117147=UNCERTAINTY_MEASURE_WITH_UNIT(LENGTH_MEASURE(0.01),#117171,
'DISTANCE_ACCURACY_VALUE',
'Maximum model space distance between geometric entities at asserted c
onnectivities') ;
#117153=(
GEOMETRIC_REPRESENTATION_CONTEXT(3)
GLOBAL_UNCERTAINTY_ASSIGNED_CONTEXT((#117130))
GLOBAL_UNIT_ASSIGNED_CONTEXT((#117171,#117173,#117174))
REPRESENTATION_CONTEXT('','3D')
) ;
#117170=(
GEOMETRIC_REPRESENTATION_CONTEXT(3)
GLOBAL_UNCERTAINTY_ASSIGNED_CONTEXT((#117147))
GLOBAL_UNIT_ASSIGNED_CONTEXT((#117171,#117173,#117174))
REPRESENTATION_CONTEXT('','3D')
) ;
#117171=(
LENGTH_UNIT()
NAMED_UNIT(*)
SI_UNIT(.MILLI.,.METRE.)
) ;
#117173=(
NAMED_UNIT(*)
PLANE_ANGLE_UNIT()
SI_UNIT($,.RADIAN.)
) ;
#117174=(
NAMED_UNIT(*)
SI_UNIT($,.STERADIAN.)
SOLID_ANGLE_UNIT()
) ;
#117180=SHAPE_DEFINITION_REPRESENTATION(#117202,#117245) ;
#117202=PRODUCT_DEFINITION_SHAPE('',$,#117268) ;
#117245=SHAPE_REPRESENTATION('',(#51734),#117153) ;
#117262=PRODUCT_DEFINITION_CONTEXT('part definition',#117330,'design') ;
#117268=PRODUCT_DEFINITION('Cover_Plate','Cover_Plate',#117290,#117262) ;
#117290=PRODUCT_DEFINITION_FORMATION('',$,#117337) ;
#117330=APPLICATION_CONTEXT(
'Core Data for Automotive Mechanical Design Process') ;
#117331=PRODUCT_CONTEXT('part definition',#117330,'mechanical') ;
#117337=PRODUCT('Cover_Plate','Cover_Plate',$,(#117331)) ;
#117355=PRESENTATION_STYLE_ASSIGNMENT((#117357)) ;
#117357=SURFACE_STYLE_USAGE(.BOTH.,#117359) ;
#117359=SURFACE_SIDE_STYLE('',(#117361)) ;
#117361=SURFACE_STYLE_FILL_AREA(#117363) ;
#117363=FILL_AREA_STYLE('Opaque(160,160,160)',(#117365)) ;
#117365=FILL_AREA_STYLE_COLOUR('Opaque(160,160,160)',#117367) ;
#117367=COLOUR_RGB('Opaque(160,160,160)', 0.09019608, 0.27058824, 0.51372549) ;
ENDSEC;
END-ISO-10303-21;
